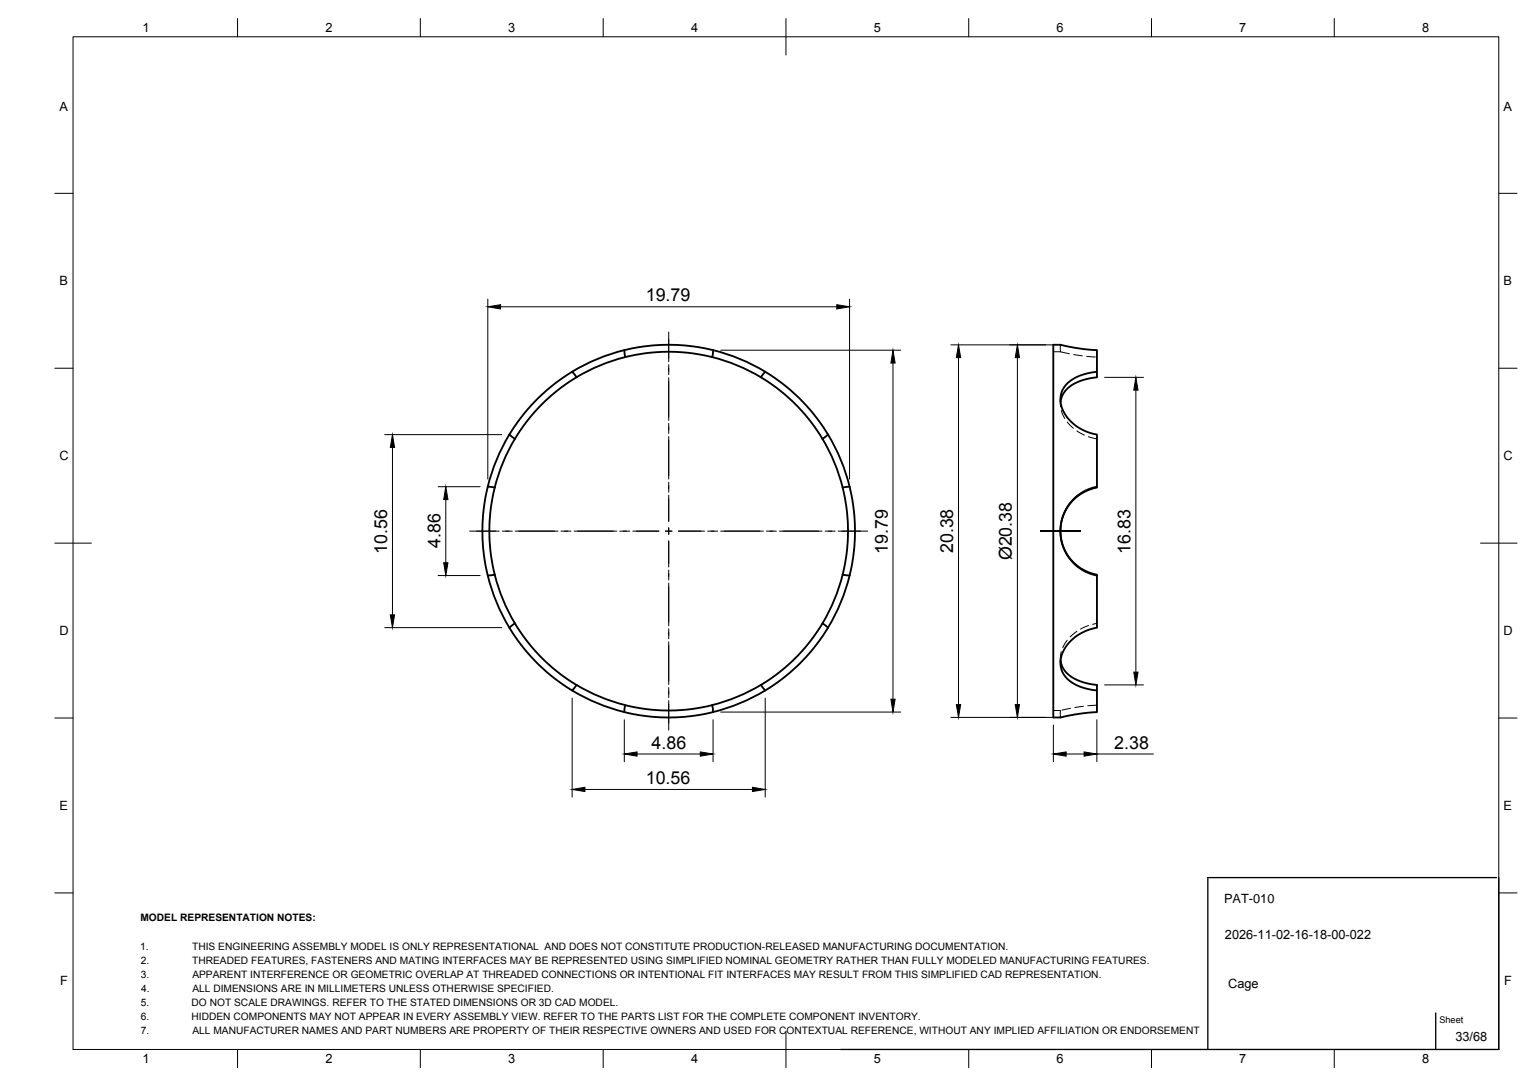
ISO-10303-21;
HEADER;
/* Generated by software containing ST-Developer
 * from STEP Tools, Inc. (www.steptools.com) 
 */

FILE_DESCRIPTION(
/* description */ ('Belt conveyor head drive unit'),
/* implementation_level */ '2;1');

FILE_NAME(
/* name */ 'Cage.step',
/* time_stamp */ '2026-10-28T03:26:19-07:00',
/* author */ (''),
/* organization */ (''),
/* preprocessor_version */ 'ST-DEVELOPER v20.2',
/* originating_system */ 'Autodesk Translation Framework v15.17.0.0',
/* authorisation */ '');

FILE_SCHEMA (('AUTOMOTIVE_DESIGN { 1 0 10303 214 3 1 1 }'));
ENDSEC;

DATA;
#10=MECHANICAL_DESIGN_GEOMETRIC_PRESENTATION_REPRESENTATION('',(#884),#27069);
#521=B_SPLINE_CURVE_WITH_KNOTS('',3,(#22504,#22505,#22506,#22507,#22508,
#22509,#22510,#22511,#22512,#22513,#22514,#22515,#22516,#22517,#22518,#22519,
#22520,#22521,#22522,#22523,#22524,#22525),.UNSPECIFIED.,.F.,.F.,(4,2,2,
2,2,2,2,2,2,2,4),(0.0473477652366656,0.126350602536658,0.189525903804987,
0.252701205073317,0.313298422430275,0.373895639787233,0.434492857144191,
0.495090074501149,0.558265375769478,0.621440677037807,0.7004435143378),
 .UNSPECIFIED.);
#522=B_SPLINE_CURVE_WITH_KNOTS('',3,(#22529,#22530,#22531,#22532,#22533,
#22534,#22535,#22536,#22537,#22538,#22539,#22540,#22541,#22542,#22543,#22544,
#22545,#22546,#22547,#22548,#22549,#22550),.UNSPECIFIED.,.F.,.F.,(4,2,2,
2,2,2,2,2,2,2,4),(0.0464897534940957,0.0852567806515119,0.170513561303024,
0.246687263103517,0.308657850341199,0.370628437578881,0.432599024816563,
0.494569612054245,0.570743313854739,0.656000094506251,0.694767121663666),
 .UNSPECIFIED.);
#523=B_SPLINE_CURVE_WITH_KNOTS('',3,(#22556,#22557,#22558,#22559,#22560,
#22561,#22562,#22563,#22564,#22565,#22566,#22567,#22568,#22569,#22570,#22571,
#22572,#22573,#22574,#22575,#22576,#22577),.UNSPECIFIED.,.F.,.F.,(4,2,2,
2,2,2,2,2,2,2,4),(0.0464897534940957,0.0852567806515118,0.170513561303024,
0.246687263103517,0.308657850341199,0.370628437578881,0.432599024816563,
0.494569612054245,0.570743313854738,0.65600009450625,0.694767121663666),
 .UNSPECIFIED.);
#524=B_SPLINE_CURVE_WITH_KNOTS('',3,(#22581,#22582,#22583,#22584,#22585,
#22586,#22587,#22588,#22589,#22590,#22591,#22592,#22593,#22594,#22595,#22596,
#22597,#22598,#22599,#22600,#22601,#22602),.UNSPECIFIED.,.F.,.F.,(4,2,2,
2,2,2,2,2,2,2,4),(0.0464897534940957,0.0852567806515119,0.170513561303024,
0.246687263103517,0.308657850341199,0.370628437578881,0.432599024816563,
0.494569612054245,0.570743313854739,0.656000094506251,0.694767121663666),
 .UNSPECIFIED.);
#525=B_SPLINE_CURVE_WITH_KNOTS('',3,(#22606,#22607,#22608,#22609,#22610,
#22611,#22612,#22613,#22614,#22615,#22616,#22617),.UNSPECIFIED.,.F.,.F.,
(4,2,2,2,2,4),(0.0464897534940957,0.0852567806515119,0.170513561303024,
0.246687263103517,0.308657850341199,0.370628437578881),.UNSPECIFIED.);
#526=B_SPLINE_CURVE_WITH_KNOTS('',3,(#22622,#22623,#22624,#22625,#22626,
#22627,#22628,#22629,#22630,#22631,#22632,#22633),.UNSPECIFIED.,.F.,.F.,
(4,2,2,2,2,4),(0.370628437578881,0.432599024816563,0.494569612054245,0.570743313854738,
0.65600009450625,0.694767121663666),.UNSPECIFIED.);
#527=B_SPLINE_CURVE_WITH_KNOTS('',3,(#22637,#22638,#22639,#22640,#22641,
#22642,#22643,#22644,#22645,#22646,#22647,#22648,#22649,#22650,#22651,#22652,
#22653,#22654,#22655,#22656,#22657,#22658),.UNSPECIFIED.,.F.,.F.,(4,2,2,
2,2,2,2,2,2,2,4),(0.0464897534940957,0.0852567806515121,0.170513561303024,
0.246687263103518,0.308657850341199,0.370628437578881,0.432599024816563,
0.494569612054245,0.570743313854738,0.65600009450625,0.694767121663666),
 .UNSPECIFIED.);
#528=B_SPLINE_CURVE_WITH_KNOTS('',3,(#22662,#22663,#22664,#22665,#22666,
#22667,#22668,#22669,#22670,#22671,#22672,#22673,#22674,#22675,#22676,#22677,
#22678,#22679,#22680,#22681,#22682,#22683),.UNSPECIFIED.,.F.,.F.,(4,2,2,
2,2,2,2,2,2,2,4),(0.0464897534940957,0.0852567806515119,0.170513561303024,
0.246687263103517,0.308657850341199,0.370628437578881,0.432599024816563,
0.494569612054245,0.570743313854738,0.65600009450625,0.694767121663667),
 .UNSPECIFIED.);
#529=B_SPLINE_CURVE_WITH_KNOTS('',3,(#22687,#22688,#22689,#22690,#22691,
#22692,#22693,#22694,#22695,#22696,#22697,#22698,#22699,#22700,#22701,#22702,
#22703,#22704,#22705,#22706,#22707,#22708),.UNSPECIFIED.,.F.,.F.,(4,2,2,
2,2,2,2,2,2,2,4),(0.0464897534940957,0.0852567806515119,0.170513561303024,
0.246687263103517,0.308657850341199,0.370628437578881,0.432599024816563,
0.494569612054245,0.570743313854738,0.65600009450625,0.694767121663666),
 .UNSPECIFIED.);
#530=B_SPLINE_CURVE_WITH_KNOTS('',3,(#22712,#22713,#22714,#22715,#22716,
#22717,#22718,#22719,#22720,#22721,#22722,#22723,#22724,#22725,#22726,#22727,
#22728,#22729,#22730,#22731,#22732,#22733),.UNSPECIFIED.,.F.,.F.,(4,2,2,
2,2,2,2,2,2,2,4),(0.0464897534940957,0.0852567806515119,0.170513561303024,
0.246687263103517,0.308657850341199,0.370628437578881,0.432599024816563,
0.494569612054245,0.570743313854739,0.656000094506251,0.694767121663667),
 .UNSPECIFIED.);
#531=B_SPLINE_CURVE_WITH_KNOTS('',3,(#22741,#22742,#22743,#22744,#22745,
#22746,#22747,#22748,#22749,#22750,#22751,#22752,#22753,#22754,#22755,#22756,
#22757,#22758,#22759,#22760,#22761,#22762),.UNSPECIFIED.,.F.,.F.,(4,2,2,
2,2,2,2,2,2,2,4),(0.0473477652366656,0.126350602536658,0.189525903804987,
0.252701205073316,0.313298422430274,0.373895639787232,0.434492857144191,
0.495090074501149,0.558265375769478,0.621440677037807,0.7004435143378),
 .UNSPECIFIED.);
#532=B_SPLINE_CURVE_WITH_KNOTS('',3,(#22770,#22771,#22772,#22773,#22774,
#22775,#22776,#22777,#22778,#22779,#22780,#22781,#22782,#22783,#22784,#22785,
#22786,#22787,#22788,#22789,#22790,#22791),.UNSPECIFIED.,.F.,.F.,(4,2,2,
2,2,2,2,2,2,2,4),(0.0473477652366656,0.126350602536658,0.189525903804987,
0.252701205073317,0.313298422430275,0.373895639787233,0.434492857144191,
0.495090074501149,0.558265375769478,0.621440677037807,0.7004435143378),
 .UNSPECIFIED.);
#533=B_SPLINE_CURVE_WITH_KNOTS('',3,(#22800,#22801,#22802,#22803,#22804,
#22805,#22806,#22807,#22808,#22809,#22810,#22811),.UNSPECIFIED.,.F.,.F.,
(4,2,2,2,2,4),(0.0473477652366656,0.126350602536658,0.189525903804987,0.252701205073316,
0.313298422430275,0.373895639787233),.UNSPECIFIED.);
#534=B_SPLINE_CURVE_WITH_KNOTS('',3,(#22813,#22814,#22815,#22816,#22817,
#22818,#22819,#22820,#22821,#22822,#22823,#22824),.UNSPECIFIED.,.F.,.F.,
(4,2,2,2,2,4),(0.373895639787233,0.434492857144191,0.495090074501149,0.558265375769478,
0.621440677037807,0.7004435143378),.UNSPECIFIED.);
#535=B_SPLINE_CURVE_WITH_KNOTS('',3,(#22831,#22832,#22833,#22834,#22835,
#22836,#22837,#22838,#22839,#22840,#22841,#22842,#22843,#22844,#22845,#22846,
#22847,#22848,#22849,#22850,#22851,#22852),.UNSPECIFIED.,.F.,.F.,(4,2,2,
2,2,2,2,2,2,2,4),(0.0473477652366656,0.126350602536658,0.189525903804987,
0.252701205073316,0.313298422430275,0.373895639787233,0.434492857144191,
0.495090074501149,0.558265375769478,0.621440677037807,0.7004435143378),
 .UNSPECIFIED.);
#536=B_SPLINE_CURVE_WITH_KNOTS('',3,(#22860,#22861,#22862,#22863,#22864,
#22865,#22866,#22867,#22868,#22869,#22870,#22871,#22872,#22873,#22874,#22875,
#22876,#22877,#22878,#22879,#22880,#22881),.UNSPECIFIED.,.F.,.F.,(4,2,2,
2,2,2,2,2,2,2,4),(0.0473477652366656,0.126350602536658,0.189525903804987,
0.252701205073317,0.313298422430275,0.373895639787233,0.434492857144191,
0.495090074501149,0.558265375769478,0.621440677037807,0.7004435143378),
 .UNSPECIFIED.);
#537=B_SPLINE_CURVE_WITH_KNOTS('',3,(#22889,#22890,#22891,#22892,#22893,
#22894,#22895,#22896,#22897,#22898,#22899,#22900,#22901,#22902,#22903,#22904,
#22905,#22906,#22907,#22908,#22909,#22910),.UNSPECIFIED.,.F.,.F.,(4,2,2,
2,2,2,2,2,2,2,4),(0.0473477652366656,0.126350602536658,0.189525903804987,
0.252701205073316,0.313298422430275,0.373895639787233,0.434492857144191,
0.495090074501149,0.558265375769478,0.621440677037807,0.7004435143378),
 .UNSPECIFIED.);
#538=B_SPLINE_CURVE_WITH_KNOTS('',3,(#22919,#22920,#22921,#22922,#22923,
#22924,#22925,#22926,#22927,#22928,#22929,#22930,#22931,#22932,#22933,#22934,
#22935,#22936,#22937,#22938,#22939,#22940),.UNSPECIFIED.,.F.,.F.,(4,2,2,
2,2,2,2,2,2,2,4),(0.0473477652366656,0.126350602536658,0.189525903804987,
0.252701205073317,0.313298422430275,0.373895639787233,0.434492857144191,
0.495090074501149,0.558265375769478,0.621440677037807,0.7004435143378),
 .UNSPECIFIED.);
#653=SPHERICAL_SURFACE('',#15248,0.247676);
#654=SPHERICAL_SURFACE('',#15264,0.247676);
#655=SPHERICAL_SURFACE('',#15269,0.247676);
#656=SPHERICAL_SURFACE('',#15274,0.247676);
#657=SPHERICAL_SURFACE('',#15279,0.247676);
#658=SPHERICAL_SURFACE('',#15284,0.247676);
#659=SPHERICAL_SURFACE('',#15289,0.247676);
#660=SPHERICAL_SURFACE('',#15297,0.247676);
#739=SHAPE_REPRESENTATION_RELATIONSHIP('SRR','None',#27384,#808);
#808=ADVANCED_BREP_SHAPE_REPRESENTATION('',(#969),#27026);
#884=STYLED_ITEM('',(#27797),#969);
#969=MANIFOLD_SOLID_BREP('Continuous crown cage',#13749);
#1155=FACE_BOUND('',#2920,.T.);
#1441=PLANE('',#15261);
#1442=PLANE('',#15266);
#1443=PLANE('',#15271);
#1444=PLANE('',#15276);
#1445=PLANE('',#15281);
#1446=PLANE('',#15286);
#1447=PLANE('',#15295);
#1448=PLANE('',#15299);
#1449=PLANE('',#15300);
#1959=FACE_OUTER_BOUND('',#2902,.T.);
#1960=FACE_OUTER_BOUND('',#2903,.T.);
#1961=FACE_OUTER_BOUND('',#2904,.T.);
#1962=FACE_OUTER_BOUND('',#2905,.T.);
#1963=FACE_OUTER_BOUND('',#2906,.T.);
#1964=FACE_OUTER_BOUND('',#2907,.T.);
#1965=FACE_OUTER_BOUND('',#2908,.T.);
#1966=FACE_OUTER_BOUND('',#2909,.T.);
#1967=FACE_OUTER_BOUND('',#2910,.T.);
#1968=FACE_OUTER_BOUND('',#2911,.T.);
#1969=FACE_OUTER_BOUND('',#2912,.T.);
#1970=FACE_OUTER_BOUND('',#2913,.T.);
#1971=FACE_OUTER_BOUND('',#2914,.T.);
#1972=FACE_OUTER_BOUND('',#2915,.T.);
#1973=FACE_OUTER_BOUND('',#2916,.T.);
#1974=FACE_OUTER_BOUND('',#2917,.T.);
#1975=FACE_OUTER_BOUND('',#2918,.T.);
#1976=FACE_OUTER_BOUND('',#2919,.T.);
#1977=FACE_OUTER_BOUND('',#2921,.T.);
#2902=EDGE_LOOP('',(#10352,#10353,#10354,#10355));
#2903=EDGE_LOOP('',(#10356,#10357,#10358,#10359,#10360,#10361,#10362,#10363,
#10364,#10365,#10366,#10367,#10368,#10369,#10370,#10371,#10372,#10373,#10374,
#10375));
#2904=EDGE_LOOP('',(#10376,#10377,#10378,#10379));
#2905=EDGE_LOOP('',(#10380,#10381,#10382,#10383));
#2906=EDGE_LOOP('',(#10384,#10385,#10386,#10387));
#2907=EDGE_LOOP('',(#10388,#10389,#10390,#10391));
#2908=EDGE_LOOP('',(#10392,#10393,#10394,#10395));
#2909=EDGE_LOOP('',(#10396,#10397,#10398,#10399,#10400,#10401));
#2910=EDGE_LOOP('',(#10402,#10403,#10404,#10405));
#2911=EDGE_LOOP('',(#10406,#10407,#10408,#10409));
#2912=EDGE_LOOP('',(#10410,#10411,#10412,#10413));
#2913=EDGE_LOOP('',(#10414,#10415,#10416,#10417));
#2914=EDGE_LOOP('',(#10418,#10419,#10420,#10421));
#2915=EDGE_LOOP('',(#10422,#10423,#10424,#10425));
#2916=EDGE_LOOP('',(#10426,#10427,#10428,#10429,#10430,#10431,#10432,#10433,
#10434,#10435,#10436,#10437,#10438,#10439,#10440,#10441,#10442,#10443,#10444,
#10445));
#2917=EDGE_LOOP('',(#10446,#10447,#10448,#10449));
#2918=EDGE_LOOP('',(#10450,#10451,#10452,#10453));
#2919=EDGE_LOOP('',(#10454));
#2920=EDGE_LOOP('',(#10455));
#2921=EDGE_LOOP('',(#10456,#10457,#10458,#10459));
#3869=LINE('',#22619,#4661);
#3870=LINE('',#22915,#4662);
#4661=VECTOR('',#18191,1.019052);
#4662=VECTOR('',#18268,0.980948);
#5408=CIRCLE('',#15249,0.243053047864041);
#5409=CIRCLE('',#15250,0.243053047864041);
#5410=CIRCLE('',#15252,1.019052);
#5411=CIRCLE('',#15253,1.019052);
#5412=CIRCLE('',#15254,1.019052);
#5413=CIRCLE('',#15255,1.019052);
#5414=CIRCLE('',#15256,1.019052);
#5415=CIRCLE('',#15257,1.019052);
#5416=CIRCLE('',#15258,1.019052);
#5417=CIRCLE('',#15259,1.019052);
#5418=CIRCLE('',#15260,1.019052);
#5419=CIRCLE('',#15262,0.980948);
#5420=CIRCLE('',#15263,0.243053047864041);
#5421=CIRCLE('',#15265,0.243053047864041);
#5422=CIRCLE('',#15267,0.980948);
#5423=CIRCLE('',#15268,0.243053047864041);
#5424=CIRCLE('',#15270,0.243053047864041);
#5425=CIRCLE('',#15272,0.980948);
#5426=CIRCLE('',#15273,0.243053047864041);
#5427=CIRCLE('',#15275,0.243053047864041);
#5428=CIRCLE('',#15277,0.980948);
#5429=CIRCLE('',#15278,0.243053047864041);
#5430=CIRCLE('',#15280,0.243053047864041);
#5431=CIRCLE('',#15282,0.980948);
#5432=CIRCLE('',#15283,0.243053047864041);
#5433=CIRCLE('',#15285,0.243053047864041);
#5434=CIRCLE('',#15287,0.980948);
#5435=CIRCLE('',#15288,0.243053047864041);
#5436=CIRCLE('',#15290,0.243053047864041);
#5437=CIRCLE('',#15292,0.980948);
#5438=CIRCLE('',#15293,0.980948);
#5439=CIRCLE('',#15294,0.980948);
#5440=CIRCLE('',#15296,0.243053047864041);
#5441=CIRCLE('',#15298,0.243053047864041);
#6427=VERTEX_POINT('',#22502);
#6428=VERTEX_POINT('',#22503);
#6429=VERTEX_POINT('',#22526);
#6430=VERTEX_POINT('',#22528);
#6431=VERTEX_POINT('',#22553);
#6432=VERTEX_POINT('',#22555);
#6433=VERTEX_POINT('',#22578);
#6434=VERTEX_POINT('',#22580);
#6435=VERTEX_POINT('',#22603);
#6436=VERTEX_POINT('',#22605);
#6437=VERTEX_POINT('',#22618);
#6438=VERTEX_POINT('',#22621);
#6439=VERTEX_POINT('',#22634);
#6440=VERTEX_POINT('',#22636);
#6441=VERTEX_POINT('',#22659);
#6442=VERTEX_POINT('',#22661);
#6443=VERTEX_POINT('',#22684);
#6444=VERTEX_POINT('',#22686);
#6445=VERTEX_POINT('',#22709);
#6446=VERTEX_POINT('',#22711);
#6447=VERTEX_POINT('',#22736);
#6448=VERTEX_POINT('',#22740);
#6449=VERTEX_POINT('',#22765);
#6450=VERTEX_POINT('',#22769);
#6451=VERTEX_POINT('',#22794);
#6452=VERTEX_POINT('',#22798);
#6453=VERTEX_POINT('',#22799);
#6454=VERTEX_POINT('',#22826);
#6455=VERTEX_POINT('',#22830);
#6456=VERTEX_POINT('',#22855);
#6457=VERTEX_POINT('',#22859);
#6458=VERTEX_POINT('',#22884);
#6459=VERTEX_POINT('',#22888);
#6460=VERTEX_POINT('',#22913);
#6461=VERTEX_POINT('',#22916);
#6462=VERTEX_POINT('',#22918);
#7868=EDGE_CURVE('',#6427,#6428,#521,.T.);
#7869=EDGE_CURVE('',#6429,#6427,#5408,.T.);
#7870=EDGE_CURVE('',#6430,#6429,#522,.T.);
#7871=EDGE_CURVE('',#6428,#6430,#5409,.T.);
#7872=EDGE_CURVE('',#6431,#6429,#5410,.T.);
#7873=EDGE_CURVE('',#6431,#6432,#523,.T.);
#7874=EDGE_CURVE('',#6433,#6432,#5411,.T.);
#7875=EDGE_CURVE('',#6433,#6434,#524,.T.);
#7876=EDGE_CURVE('',#6435,#6434,#5412,.T.);
#7877=EDGE_CURVE('',#6435,#6436,#525,.T.);
#7878=EDGE_CURVE('',#6436,#6437,#3869,.T.);
#7879=EDGE_CURVE('',#6437,#6437,#5413,.T.);
#7880=EDGE_CURVE('',#6436,#6438,#526,.T.);
#7881=EDGE_CURVE('',#6439,#6438,#5414,.T.);
#7882=EDGE_CURVE('',#6439,#6440,#527,.T.);
#7883=EDGE_CURVE('',#6441,#6440,#5415,.T.);
#7884=EDGE_CURVE('',#6441,#6442,#528,.T.);
#7885=EDGE_CURVE('',#6443,#6442,#5416,.T.);
#7886=EDGE_CURVE('',#6443,#6444,#529,.T.);
#7887=EDGE_CURVE('',#6445,#6444,#5417,.T.);
#7888=EDGE_CURVE('',#6445,#6446,#530,.T.);
#7889=EDGE_CURVE('',#6430,#6446,#5418,.T.);
#7890=EDGE_CURVE('',#6427,#6447,#5419,.T.);
#7891=EDGE_CURVE('',#6447,#6431,#5420,.T.);
#7892=EDGE_CURVE('',#6448,#6447,#531,.T.);
#7893=EDGE_CURVE('',#6432,#6448,#5421,.T.);
#7894=EDGE_CURVE('',#6448,#6449,#5422,.T.);
#7895=EDGE_CURVE('',#6449,#6433,#5423,.T.);
#7896=EDGE_CURVE('',#6450,#6449,#532,.T.);
#7897=EDGE_CURVE('',#6434,#6450,#5424,.T.);
#7898=EDGE_CURVE('',#6450,#6451,#5425,.T.);
#7899=EDGE_CURVE('',#6451,#6435,#5426,.T.);
#7900=EDGE_CURVE('',#6452,#6453,#533,.T.);
#7901=EDGE_CURVE('',#6438,#6452,#5427,.T.);
#7902=EDGE_CURVE('',#6453,#6451,#534,.T.);
#7903=EDGE_CURVE('',#6452,#6454,#5428,.T.);
#7904=EDGE_CURVE('',#6454,#6439,#5429,.T.);
#7905=EDGE_CURVE('',#6455,#6454,#535,.T.);
#7906=EDGE_CURVE('',#6440,#6455,#5430,.T.);
#7907=EDGE_CURVE('',#6455,#6456,#5431,.T.);
#7908=EDGE_CURVE('',#6456,#6441,#5432,.T.);
#7909=EDGE_CURVE('',#6457,#6456,#536,.T.);
#7910=EDGE_CURVE('',#6442,#6457,#5433,.T.);
#7911=EDGE_CURVE('',#6457,#6458,#5434,.T.);
#7912=EDGE_CURVE('',#6458,#6443,#5435,.T.);
#7913=EDGE_CURVE('',#6459,#6458,#537,.T.);
#7914=EDGE_CURVE('',#6444,#6459,#5436,.T.);
#7915=EDGE_CURVE('',#6460,#6460,#5437,.T.);
#7916=EDGE_CURVE('',#6460,#6453,#3870,.T.);
#7917=EDGE_CURVE('',#6461,#6428,#5438,.T.);
#7918=EDGE_CURVE('',#6461,#6462,#538,.T.);
#7919=EDGE_CURVE('',#6459,#6462,#5439,.T.);
#7920=EDGE_CURVE('',#6446,#6461,#5440,.T.);
#7921=EDGE_CURVE('',#6462,#6445,#5441,.T.);
#10352=ORIENTED_EDGE('',*,*,#7868,.F.);
#10353=ORIENTED_EDGE('',*,*,#7869,.F.);
#10354=ORIENTED_EDGE('',*,*,#7870,.F.);
#10355=ORIENTED_EDGE('',*,*,#7871,.F.);
#10356=ORIENTED_EDGE('',*,*,#7870,.T.);
#10357=ORIENTED_EDGE('',*,*,#7872,.F.);
#10358=ORIENTED_EDGE('',*,*,#7873,.T.);
#10359=ORIENTED_EDGE('',*,*,#7874,.F.);
#10360=ORIENTED_EDGE('',*,*,#7875,.T.);
#10361=ORIENTED_EDGE('',*,*,#7876,.F.);
#10362=ORIENTED_EDGE('',*,*,#7877,.T.);
#10363=ORIENTED_EDGE('',*,*,#7878,.T.);
#10364=ORIENTED_EDGE('',*,*,#7879,.F.);
#10365=ORIENTED_EDGE('',*,*,#7878,.F.);
#10366=ORIENTED_EDGE('',*,*,#7880,.T.);
#10367=ORIENTED_EDGE('',*,*,#7881,.F.);
#10368=ORIENTED_EDGE('',*,*,#7882,.T.);
#10369=ORIENTED_EDGE('',*,*,#7883,.F.);
#10370=ORIENTED_EDGE('',*,*,#7884,.T.);
#10371=ORIENTED_EDGE('',*,*,#7885,.F.);
#10372=ORIENTED_EDGE('',*,*,#7886,.T.);
#10373=ORIENTED_EDGE('',*,*,#7887,.F.);
#10374=ORIENTED_EDGE('',*,*,#7888,.T.);
#10375=ORIENTED_EDGE('',*,*,#7889,.F.);
#10376=ORIENTED_EDGE('',*,*,#7869,.T.);
#10377=ORIENTED_EDGE('',*,*,#7890,.T.);
#10378=ORIENTED_EDGE('',*,*,#7891,.T.);
#10379=ORIENTED_EDGE('',*,*,#7872,.T.);
#10380=ORIENTED_EDGE('',*,*,#7892,.F.);
#10381=ORIENTED_EDGE('',*,*,#7893,.F.);
#10382=ORIENTED_EDGE('',*,*,#7873,.F.);
#10383=ORIENTED_EDGE('',*,*,#7891,.F.);
#10384=ORIENTED_EDGE('',*,*,#7893,.T.);
#10385=ORIENTED_EDGE('',*,*,#7894,.T.);
#10386=ORIENTED_EDGE('',*,*,#7895,.T.);
#10387=ORIENTED_EDGE('',*,*,#7874,.T.);
#10388=ORIENTED_EDGE('',*,*,#7896,.F.);
#10389=ORIENTED_EDGE('',*,*,#7897,.F.);
#10390=ORIENTED_EDGE('',*,*,#7875,.F.);
#10391=ORIENTED_EDGE('',*,*,#7895,.F.);
#10392=ORIENTED_EDGE('',*,*,#7897,.T.);
#10393=ORIENTED_EDGE('',*,*,#7898,.T.);
#10394=ORIENTED_EDGE('',*,*,#7899,.T.);
#10395=ORIENTED_EDGE('',*,*,#7876,.T.);
#10396=ORIENTED_EDGE('',*,*,#7900,.F.);
#10397=ORIENTED_EDGE('',*,*,#7901,.F.);
#10398=ORIENTED_EDGE('',*,*,#7880,.F.);
#10399=ORIENTED_EDGE('',*,*,#7877,.F.);
#10400=ORIENTED_EDGE('',*,*,#7899,.F.);
#10401=ORIENTED_EDGE('',*,*,#7902,.F.);
#10402=ORIENTED_EDGE('',*,*,#7901,.T.);
#10403=ORIENTED_EDGE('',*,*,#7903,.T.);
#10404=ORIENTED_EDGE('',*,*,#7904,.T.);
#10405=ORIENTED_EDGE('',*,*,#7881,.T.);
#10406=ORIENTED_EDGE('',*,*,#7905,.F.);
#10407=ORIENTED_EDGE('',*,*,#7906,.F.);
#10408=ORIENTED_EDGE('',*,*,#7882,.F.);
#10409=ORIENTED_EDGE('',*,*,#7904,.F.);
#10410=ORIENTED_EDGE('',*,*,#7906,.T.);
#10411=ORIENTED_EDGE('',*,*,#7907,.T.);
#10412=ORIENTED_EDGE('',*,*,#7908,.T.);
#10413=ORIENTED_EDGE('',*,*,#7883,.T.);
#10414=ORIENTED_EDGE('',*,*,#7909,.F.);
#10415=ORIENTED_EDGE('',*,*,#7910,.F.);
#10416=ORIENTED_EDGE('',*,*,#7884,.F.);
#10417=ORIENTED_EDGE('',*,*,#7908,.F.);
#10418=ORIENTED_EDGE('',*,*,#7910,.T.);
#10419=ORIENTED_EDGE('',*,*,#7911,.T.);
#10420=ORIENTED_EDGE('',*,*,#7912,.T.);
#10421=ORIENTED_EDGE('',*,*,#7885,.T.);
#10422=ORIENTED_EDGE('',*,*,#7886,.F.);
#10423=ORIENTED_EDGE('',*,*,#7912,.F.);
#10424=ORIENTED_EDGE('',*,*,#7913,.F.);
#10425=ORIENTED_EDGE('',*,*,#7914,.F.);
#10426=ORIENTED_EDGE('',*,*,#7915,.F.);
#10427=ORIENTED_EDGE('',*,*,#7916,.T.);
#10428=ORIENTED_EDGE('',*,*,#7902,.T.);
#10429=ORIENTED_EDGE('',*,*,#7898,.F.);
#10430=ORIENTED_EDGE('',*,*,#7896,.T.);
#10431=ORIENTED_EDGE('',*,*,#7894,.F.);
#10432=ORIENTED_EDGE('',*,*,#7892,.T.);
#10433=ORIENTED_EDGE('',*,*,#7890,.F.);
#10434=ORIENTED_EDGE('',*,*,#7868,.T.);
#10435=ORIENTED_EDGE('',*,*,#7917,.F.);
#10436=ORIENTED_EDGE('',*,*,#7918,.T.);
#10437=ORIENTED_EDGE('',*,*,#7919,.F.);
#10438=ORIENTED_EDGE('',*,*,#7913,.T.);
#10439=ORIENTED_EDGE('',*,*,#7911,.F.);
#10440=ORIENTED_EDGE('',*,*,#7909,.T.);
#10441=ORIENTED_EDGE('',*,*,#7907,.F.);
#10442=ORIENTED_EDGE('',*,*,#7905,.T.);
#10443=ORIENTED_EDGE('',*,*,#7903,.F.);
#10444=ORIENTED_EDGE('',*,*,#7900,.T.);
#10445=ORIENTED_EDGE('',*,*,#7916,.F.);
#10446=ORIENTED_EDGE('',*,*,#7871,.T.);
#10447=ORIENTED_EDGE('',*,*,#7889,.T.);
#10448=ORIENTED_EDGE('',*,*,#7920,.T.);
#10449=ORIENTED_EDGE('',*,*,#7917,.T.);
#10450=ORIENTED_EDGE('',*,*,#7888,.F.);
#10451=ORIENTED_EDGE('',*,*,#7921,.F.);
#10452=ORIENTED_EDGE('',*,*,#7918,.F.);
#10453=ORIENTED_EDGE('',*,*,#7920,.F.);
#10454=ORIENTED_EDGE('',*,*,#7879,.T.);
#10455=ORIENTED_EDGE('',*,*,#7915,.T.);
#10456=ORIENTED_EDGE('',*,*,#7914,.T.);
#10457=ORIENTED_EDGE('',*,*,#7919,.T.);
#10458=ORIENTED_EDGE('',*,*,#7921,.T.);
#10459=ORIENTED_EDGE('',*,*,#7887,.T.);
#12680=CYLINDRICAL_SURFACE('',#15251,1.019052);
#12681=CYLINDRICAL_SURFACE('',#15291,0.980948);
#13238=ADVANCED_FACE('',(#1959),#653,.F.);
#13239=ADVANCED_FACE('',(#1960),#12680,.T.);
#13240=ADVANCED_FACE('',(#1961),#1441,.T.);
#13241=ADVANCED_FACE('',(#1962),#654,.F.);
#13242=ADVANCED_FACE('',(#1963),#1442,.T.);
#13243=ADVANCED_FACE('',(#1964),#655,.F.);
#13244=ADVANCED_FACE('',(#1965),#1443,.T.);
#13245=ADVANCED_FACE('',(#1966),#656,.F.);
#13246=ADVANCED_FACE('',(#1967),#1444,.T.);
#13247=ADVANCED_FACE('',(#1968),#657,.F.);
#13248=ADVANCED_FACE('',(#1969),#1445,.T.);
#13249=ADVANCED_FACE('',(#1970),#658,.F.);
#13250=ADVANCED_FACE('',(#1971),#1446,.T.);
#13251=ADVANCED_FACE('',(#1972),#659,.F.);
#13252=ADVANCED_FACE('',(#1973),#12681,.F.);
#13253=ADVANCED_FACE('',(#1974),#1447,.T.);
#13254=ADVANCED_FACE('',(#1975),#660,.F.);
#13255=ADVANCED_FACE('',(#1976,#1155),#1448,.T.);
#13256=ADVANCED_FACE('',(#1977),#1449,.T.);
#13749=CLOSED_SHELL('',(#13238,#13239,#13240,#13241,#13242,#13243,#13244,
#13245,#13246,#13247,#13248,#13249,#13250,#13251,#13252,#13253,#13254,#13255,
#13256));
#15247=AXIS2_PLACEMENT_3D('',#22500,#18175,#18176);
#15248=AXIS2_PLACEMENT_3D('',#22501,#18177,#18178);
#15249=AXIS2_PLACEMENT_3D('',#22527,#18179,#18180);
#15250=AXIS2_PLACEMENT_3D('',#22551,#18181,#18182);
#15251=AXIS2_PLACEMENT_3D('',#22552,#18183,#18184);
#15252=AXIS2_PLACEMENT_3D('',#22554,#18185,#18186);
#15253=AXIS2_PLACEMENT_3D('',#22579,#18187,#18188);
#15254=AXIS2_PLACEMENT_3D('',#22604,#18189,#18190);
#15255=AXIS2_PLACEMENT_3D('',#22620,#18192,#18193);
#15256=AXIS2_PLACEMENT_3D('',#22635,#18194,#18195);
#15257=AXIS2_PLACEMENT_3D('',#22660,#18196,#18197);
#15258=AXIS2_PLACEMENT_3D('',#22685,#18198,#18199);
#15259=AXIS2_PLACEMENT_3D('',#22710,#18200,#18201);
#15260=AXIS2_PLACEMENT_3D('',#22734,#18202,#18203);
#15261=AXIS2_PLACEMENT_3D('',#22735,#18204,#18205);
#15262=AXIS2_PLACEMENT_3D('',#22737,#18206,#18207);
#15263=AXIS2_PLACEMENT_3D('',#22738,#18208,#18209);
#15264=AXIS2_PLACEMENT_3D('',#22739,#18210,#18211);
#15265=AXIS2_PLACEMENT_3D('',#22763,#18212,#18213);
#15266=AXIS2_PLACEMENT_3D('',#22764,#18214,#18215);
#15267=AXIS2_PLACEMENT_3D('',#22766,#18216,#18217);
#15268=AXIS2_PLACEMENT_3D('',#22767,#18218,#18219);
#15269=AXIS2_PLACEMENT_3D('',#22768,#18220,#18221);
#15270=AXIS2_PLACEMENT_3D('',#22792,#18222,#18223);
#15271=AXIS2_PLACEMENT_3D('',#22793,#18224,#18225);
#15272=AXIS2_PLACEMENT_3D('',#22795,#18226,#18227);
#15273=AXIS2_PLACEMENT_3D('',#22796,#18228,#18229);
#15274=AXIS2_PLACEMENT_3D('',#22797,#18230,#18231);
#15275=AXIS2_PLACEMENT_3D('',#22812,#18232,#18233);
#15276=AXIS2_PLACEMENT_3D('',#22825,#18234,#18235);
#15277=AXIS2_PLACEMENT_3D('',#22827,#18236,#18237);
#15278=AXIS2_PLACEMENT_3D('',#22828,#18238,#18239);
#15279=AXIS2_PLACEMENT_3D('',#22829,#18240,#18241);
#15280=AXIS2_PLACEMENT_3D('',#22853,#18242,#18243);
#15281=AXIS2_PLACEMENT_3D('',#22854,#18244,#18245);
#15282=AXIS2_PLACEMENT_3D('',#22856,#18246,#18247);
#15283=AXIS2_PLACEMENT_3D('',#22857,#18248,#18249);
#15284=AXIS2_PLACEMENT_3D('',#22858,#18250,#18251);
#15285=AXIS2_PLACEMENT_3D('',#22882,#18252,#18253);
#15286=AXIS2_PLACEMENT_3D('',#22883,#18254,#18255);
#15287=AXIS2_PLACEMENT_3D('',#22885,#18256,#18257);
#15288=AXIS2_PLACEMENT_3D('',#22886,#18258,#18259);
#15289=AXIS2_PLACEMENT_3D('',#22887,#18260,#18261);
#15290=AXIS2_PLACEMENT_3D('',#22911,#18262,#18263);
#15291=AXIS2_PLACEMENT_3D('',#22912,#18264,#18265);
#15292=AXIS2_PLACEMENT_3D('',#22914,#18266,#18267);
#15293=AXIS2_PLACEMENT_3D('',#22917,#18269,#18270);
#15294=AXIS2_PLACEMENT_3D('',#22941,#18271,#18272);
#15295=AXIS2_PLACEMENT_3D('',#22942,#18273,#18274);
#15296=AXIS2_PLACEMENT_3D('',#22943,#18275,#18276);
#15297=AXIS2_PLACEMENT_3D('',#22944,#18277,#18278);
#15298=AXIS2_PLACEMENT_3D('',#22945,#18279,#18280);
#15299=AXIS2_PLACEMENT_3D('',#22946,#18281,#18282);
#15300=AXIS2_PLACEMENT_3D('',#22947,#18283,#18284);
#18175=DIRECTION('axis',(0.,0.,1.));
#18176=DIRECTION('refdir',(1.,0.,0.));
#18177=DIRECTION('center_axis',(0.,0.,1.));
#18178=DIRECTION('ref_axis',(1.,0.,0.));
#18179=DIRECTION('center_axis',(0.,-1.,0.));
#18180=DIRECTION('ref_axis',(0.,0.,-1.));
#18181=DIRECTION('center_axis',(0.,-1.,0.));
#18182=DIRECTION('ref_axis',(0.,0.,-1.));
#18183=DIRECTION('center_axis',(0.,1.,0.));
#18184=DIRECTION('ref_axis',(1.,0.,0.));
#18185=DIRECTION('center_axis',(0.,1.,0.));
#18186=DIRECTION('ref_axis',(1.,0.,0.));
#18187=DIRECTION('center_axis',(0.,1.,0.));
#18188=DIRECTION('ref_axis',(1.,0.,0.));
#18189=DIRECTION('center_axis',(0.,1.,0.));
#18190=DIRECTION('ref_axis',(1.,0.,0.));
#18191=DIRECTION('',(0.,-1.,0.));
#18192=DIRECTION('center_axis',(0.,-1.,0.));
#18193=DIRECTION('ref_axis',(1.,0.,0.));
#18194=DIRECTION('center_axis',(0.,1.,0.));
#18195=DIRECTION('ref_axis',(1.,0.,0.));
#18196=DIRECTION('center_axis',(0.,1.,0.));
#18197=DIRECTION('ref_axis',(1.,0.,0.));
#18198=DIRECTION('center_axis',(0.,1.,0.));
#18199=DIRECTION('ref_axis',(1.,0.,0.));
#18200=DIRECTION('center_axis',(0.,1.,0.));
#18201=DIRECTION('ref_axis',(1.,0.,0.));
#18202=DIRECTION('center_axis',(0.,1.,0.));
#18203=DIRECTION('ref_axis',(1.,0.,0.));
#18204=DIRECTION('center_axis',(0.,1.,0.));
#18205=DIRECTION('ref_axis',(1.,0.,0.));
#18206=DIRECTION('center_axis',(0.,-1.,0.));
#18207=DIRECTION('ref_axis',(1.,0.,0.));
#18208=DIRECTION('center_axis',(0.,-1.,0.));
#18209=DIRECTION('ref_axis',(0.,0.,-1.));
#18210=DIRECTION('center_axis',(6.12323399573677E-17,0.,1.));
#18211=DIRECTION('ref_axis',(1.,0.,0.));
#18212=DIRECTION('center_axis',(0.,-1.,0.));
#18213=DIRECTION('ref_axis',(0.,0.,-1.));
#18214=DIRECTION('center_axis',(0.,1.,0.));
#18215=DIRECTION('ref_axis',(1.,0.,0.));
#18216=DIRECTION('center_axis',(0.,-1.,0.));
#18217=DIRECTION('ref_axis',(1.,0.,0.));
#18218=DIRECTION('center_axis',(0.,-1.,0.));
#18219=DIRECTION('ref_axis',(0.,0.,-1.));
#18220=DIRECTION('center_axis',(0.,0.,1.));
#18221=DIRECTION('ref_axis',(1.,0.,0.));
#18222=DIRECTION('center_axis',(0.,-1.,0.));
#18223=DIRECTION('ref_axis',(0.,0.,-1.));
#18224=DIRECTION('center_axis',(0.,1.,0.));
#18225=DIRECTION('ref_axis',(1.,0.,0.));
#18226=DIRECTION('center_axis',(0.,-1.,0.));
#18227=DIRECTION('ref_axis',(1.,0.,0.));
#18228=DIRECTION('center_axis',(0.,-1.,0.));
#18229=DIRECTION('ref_axis',(0.,0.,-1.));
#18230=DIRECTION('center_axis',(0.,0.,1.));
#18231=DIRECTION('ref_axis',(1.,0.,0.));
#18232=DIRECTION('center_axis',(0.,-1.,0.));
#18233=DIRECTION('ref_axis',(0.,0.,-1.));
#18234=DIRECTION('center_axis',(0.,1.,0.));
#18235=DIRECTION('ref_axis',(1.,0.,0.));
#18236=DIRECTION('center_axis',(0.,-1.,0.));
#18237=DIRECTION('ref_axis',(1.,0.,0.));
#18238=DIRECTION('center_axis',(0.,-1.,0.));
#18239=DIRECTION('ref_axis',(0.,0.,-1.));
#18240=DIRECTION('center_axis',(0.,0.,1.));
#18241=DIRECTION('ref_axis',(1.,0.,0.));
#18242=DIRECTION('center_axis',(0.,-1.,0.));
#18243=DIRECTION('ref_axis',(0.,0.,-1.));
#18244=DIRECTION('center_axis',(0.,1.,0.));
#18245=DIRECTION('ref_axis',(1.,0.,0.));
#18246=DIRECTION('center_axis',(0.,-1.,0.));
#18247=DIRECTION('ref_axis',(1.,0.,0.));
#18248=DIRECTION('center_axis',(0.,-1.,0.));
#18249=DIRECTION('ref_axis',(0.,0.,-1.));
#18250=DIRECTION('center_axis',(6.12323399573676E-17,0.,1.));
#18251=DIRECTION('ref_axis',(1.,0.,0.));
#18252=DIRECTION('center_axis',(0.,-1.,0.));
#18253=DIRECTION('ref_axis',(0.,0.,-1.));
#18254=DIRECTION('center_axis',(0.,1.,0.));
#18255=DIRECTION('ref_axis',(1.,0.,0.));
#18256=DIRECTION('center_axis',(0.,-1.,0.));
#18257=DIRECTION('ref_axis',(1.,0.,0.));
#18258=DIRECTION('center_axis',(0.,-1.,0.));
#18259=DIRECTION('ref_axis',(0.,0.,-1.));
#18260=DIRECTION('center_axis',(0.,0.,1.));
#18261=DIRECTION('ref_axis',(1.,0.,0.));
#18262=DIRECTION('center_axis',(0.,-1.,0.));
#18263=DIRECTION('ref_axis',(0.,0.,-1.));
#18264=DIRECTION('center_axis',(0.,1.,0.));
#18265=DIRECTION('ref_axis',(1.,0.,0.));
#18266=DIRECTION('center_axis',(0.,1.,0.));
#18267=DIRECTION('ref_axis',(1.,0.,0.));
#18268=DIRECTION('',(0.,1.,0.));
#18269=DIRECTION('center_axis',(0.,-1.,0.));
#18270=DIRECTION('ref_axis',(1.,0.,0.));
#18271=DIRECTION('center_axis',(0.,-1.,0.));
#18272=DIRECTION('ref_axis',(1.,0.,0.));
#18273=DIRECTION('center_axis',(0.,1.,0.));
#18274=DIRECTION('ref_axis',(1.,0.,0.));
#18275=DIRECTION('center_axis',(0.,-1.,0.));
#18276=DIRECTION('ref_axis',(0.,0.,-1.));
#18277=DIRECTION('center_axis',(0.,0.,1.));
#18278=DIRECTION('ref_axis',(1.,0.,0.));
#18279=DIRECTION('center_axis',(0.,-1.,0.));
#18280=DIRECTION('ref_axis',(0.,0.,-1.));
#18281=DIRECTION('center_axis',(0.,-1.,0.));
#18282=DIRECTION('ref_axis',(-1.,0.,0.));
#18283=DIRECTION('center_axis',(0.,1.,0.));
#18284=DIRECTION('ref_axis',(1.,0.,0.));
#22500=CARTESIAN_POINT('',(0.,0.,0.));
#22501=CARTESIAN_POINT('Origin',(0.707106781186547,0.,0.707106781186548));
#22502=CARTESIAN_POINT('',(0.504455939115715,-0.04763,0.841298510752802));
#22503=CARTESIAN_POINT('',(0.841298510752802,-0.04763,0.504455939115715));
#22504=CARTESIAN_POINT('Ctrl Pts',(0.504455939115715,-0.04763,0.841298510752802));
#22505=CARTESIAN_POINT('Ctrl Pts',(0.508899795931835,-0.0740444353928835,
0.838633903678357));
#22506=CARTESIAN_POINT('Ctrl Pts',(0.517157748491652,-0.0999305678883309,
0.833661031856294));
#22507=CARTESIAN_POINT('Ctrl Pts',(0.537715343527944,-0.142345102874864,
0.820511285096538));
#22508=CARTESIAN_POINT('Ctrl Pts',(0.548874290046456,-0.159766064500479,
0.813159949759));
#22509=CARTESIAN_POINT('Ctrl Pts',(0.573915184558107,-0.190326085855194,
0.795684265985089));
#22510=CARTESIAN_POINT('Ctrl Pts',(0.587792702767295,-0.203463743702801,
0.78555112003688));
#22511=CARTESIAN_POINT('Ctrl Pts',(0.615966552324775,-0.224161999508995,
0.763642258217233));
#22512=CARTESIAN_POINT('Ctrl Pts',(0.631684198665438,-0.232861760990032,
0.750785745543687));
#22513=CARTESIAN_POINT('Ctrl Pts',(0.663382628119203,-0.244251601209411,
0.722929908501543));
#22514=CARTESIAN_POINT('Ctrl Pts',(0.679352081686668,-0.246942143572133,
0.707917883896095));
#22515=CARTESIAN_POINT('Ctrl Pts',(0.707917883896095,-0.246942143572133,
0.679352081686668));
#22516=CARTESIAN_POINT('Ctrl Pts',(0.722929908501543,-0.244251601209411,
0.663382628119203));
#22517=CARTESIAN_POINT('Ctrl Pts',(0.750785745543687,-0.232861760990032,
0.631684198665439));
#22518=CARTESIAN_POINT('Ctrl Pts',(0.763642258217232,-0.224161999508995,
0.615966552324775));
#22519=CARTESIAN_POINT('Ctrl Pts',(0.78555112003688,-0.203463743702801,
0.587792702767295));
#22520=CARTESIAN_POINT('Ctrl Pts',(0.795684265985088,-0.190326085855194,
0.573915184558108));
#22521=CARTESIAN_POINT('Ctrl Pts',(0.813159949759,-0.15976606450048,0.548874290046456));
#22522=CARTESIAN_POINT('Ctrl Pts',(0.820511285096538,-0.142345102874864,
0.537715343527944));
#22523=CARTESIAN_POINT('Ctrl Pts',(0.833661031856294,-0.099930567888331,
0.517157748491653));
#22524=CARTESIAN_POINT('Ctrl Pts',(0.838633903678357,-0.0740444353928835,
0.508899795931835));
#22525=CARTESIAN_POINT('Ctrl Pts',(0.841298510752801,-0.0476299999999999,
0.504455939115715));
#22526=CARTESIAN_POINT('',(0.528110872004958,-0.04763,0.871530771444223));
#22527=CARTESIAN_POINT('Origin',(0.707106781186547,-0.04763,0.707106781186548));
#22528=CARTESIAN_POINT('',(0.871530771444223,-0.04763,0.528110872004959));
#22529=CARTESIAN_POINT('Ctrl Pts',(0.871530771444223,-0.0476300000000001,
0.528110872004958));
#22530=CARTESIAN_POINT('Ctrl Pts',(0.87014664509073,-0.0609922781173483,
0.530395067942936));
#22531=CARTESIAN_POINT('Ctrl Pts',(0.868149331745851,-0.0742967091364493,
0.533674141594226));
#22532=CARTESIAN_POINT('Ctrl Pts',(0.85981294420286,-0.115492077056649,
0.54708917182331));
#22533=CARTESIAN_POINT('Ctrl Pts',(0.850993704737257,-0.141695629206859,
0.560922177770136));
#22534=CARTESIAN_POINT('Ctrl Pts',(0.830754510485543,-0.181890537957859,
0.590422647829571));
#22535=CARTESIAN_POINT('Ctrl Pts',(0.816896541396381,-0.201072148666545,
0.609616703125488));
#22536=CARTESIAN_POINT('Ctrl Pts',(0.792310597819928,-0.223955109275652,
0.641117951819998));
#22537=CARTESIAN_POINT('Ctrl Pts',(0.779109323683612,-0.232742381310829,
0.657208095763053));
#22538=CARTESIAN_POINT('Ctrl Pts',(0.750552691816206,-0.244234834628584,
0.68964083160521));
#22539=CARTESIAN_POINT('Ctrl Pts',(0.735185187071673,-0.246942143572133,
0.705971972091755));
#22540=CARTESIAN_POINT('Ctrl Pts',(0.705971972091754,-0.246942143572133,
0.735185187071673));
#22541=CARTESIAN_POINT('Ctrl Pts',(0.689640831605209,-0.244234834628584,
0.750552691816206));
#22542=CARTESIAN_POINT('Ctrl Pts',(0.657208095763052,-0.232742381310829,
0.779109323683612));
#22543=CARTESIAN_POINT('Ctrl Pts',(0.641117951819998,-0.223955109275652,
0.792310597819928));
#22544=CARTESIAN_POINT('Ctrl Pts',(0.609616703125487,-0.201072148666545,
0.816896541396382));
#22545=CARTESIAN_POINT('Ctrl Pts',(0.590422647829571,-0.181890537957858,
0.830754510485544));
#22546=CARTESIAN_POINT('Ctrl Pts',(0.560922177770135,-0.141695629206858,
0.850993704737257));
#22547=CARTESIAN_POINT('Ctrl Pts',(0.547089171823309,-0.115492077056649,
0.859812944202861));
#22548=CARTESIAN_POINT('Ctrl Pts',(0.533674141594226,-0.0742967091364491,
0.868149331745852));
#22549=CARTESIAN_POINT('Ctrl Pts',(0.530395067942936,-0.0609922781173483,
0.870146645090731));
#22550=CARTESIAN_POINT('Ctrl Pts',(0.528110872004958,-0.0476300000000001,
0.871530771444223));
#22551=CARTESIAN_POINT('Origin',(0.707106781186547,-0.04763,0.707106781186548));
#22552=CARTESIAN_POINT('Origin',(0.,-0.166705,0.));
#22553=CARTESIAN_POINT('',(0.242834539687906,-0.04763,0.989696097314));
#22554=CARTESIAN_POINT('Origin',(0.,-0.04763,0.));
#22555=CARTESIAN_POINT('',(-0.242834539687907,-0.04763,0.989696097314));
#22556=CARTESIAN_POINT('Ctrl Pts',(0.242834539687906,-0.04763,0.989696097314));
#22557=CARTESIAN_POINT('Ctrl Pts',(0.24024064412003,-0.0609922781173483,
0.990332542620729));
#22558=CARTESIAN_POINT('Ctrl Pts',(0.236509675094874,-0.0742967091364492,
0.991238884025248));
#22559=CARTESIAN_POINT('Ctrl Pts',(0.221129100087819,-0.115492077056649,
0.994830026707808));
#22560=CARTESIAN_POINT('Ctrl Pts',(0.205111543747588,-0.141695629206859,
0.998375294985966));
#22561=CARTESIAN_POINT('Ctrl Pts',(0.169940289819232,-0.181890537957859,
1.00492400591205));
#22562=CARTESIAN_POINT('Ctrl Pts',(0.1465689792446,-0.201072148666545,1.00869718865384));
#22563=CARTESIAN_POINT('Ctrl Pts',(0.106909345252087,-0.223955109275652,
1.01358704779679));
#22564=CARTESIAN_POINT('Ctrl Pts',(0.0861971848975941,-0.232742381310829,
1.0156297872271));
#22565=CARTESIAN_POINT('Ctrl Pts',(0.0430711894098822,-0.244234834628584,
1.01837060663223));
#22566=CARTESIAN_POINT('Ctrl Pts',(0.0206568624125605,-0.246942143572133,
1.019052));
#22567=CARTESIAN_POINT('Ctrl Pts',(-0.0206568624125608,-0.246942143572133,
1.019052));
#22568=CARTESIAN_POINT('Ctrl Pts',(-0.0430711894098825,-0.244234834628584,
1.01837060663223));
#22569=CARTESIAN_POINT('Ctrl Pts',(-0.0861971848975943,-0.232742381310829,
1.0156297872271));
#22570=CARTESIAN_POINT('Ctrl Pts',(-0.106909345252088,-0.223955109275652,
1.01358704779679));
#22571=CARTESIAN_POINT('Ctrl Pts',(-0.1465689792446,-0.201072148666545,
1.00869718865384));
#22572=CARTESIAN_POINT('Ctrl Pts',(-0.169940289819232,-0.181890537957859,
1.00492400591205));
#22573=CARTESIAN_POINT('Ctrl Pts',(-0.205111543747588,-0.141695629206859,
0.998375294985966));
#22574=CARTESIAN_POINT('Ctrl Pts',(-0.221129100087819,-0.115492077056649,
0.994830026707808));
#22575=CARTESIAN_POINT('Ctrl Pts',(-0.236509675094875,-0.0742967091364493,
0.991238884025248));
#22576=CARTESIAN_POINT('Ctrl Pts',(-0.24024064412003,-0.0609922781173483,
0.990332542620729));
#22577=CARTESIAN_POINT('Ctrl Pts',(-0.242834539687907,-0.04763,0.989696097314));
#22578=CARTESIAN_POINT('',(-0.528110872004959,-0.04763,0.871530771444223));
#22579=CARTESIAN_POINT('Origin',(0.,-0.04763,0.));
#22580=CARTESIAN_POINT('',(-0.871530771444223,-0.04763,0.528110872004958));
#22581=CARTESIAN_POINT('Ctrl Pts',(-0.528110872004958,-0.0476300000000001,
0.871530771444223));
#22582=CARTESIAN_POINT('Ctrl Pts',(-0.530395067942936,-0.0609922781173484,
0.87014664509073));
#22583=CARTESIAN_POINT('Ctrl Pts',(-0.533674141594226,-0.0742967091364493,
0.868149331745851));
#22584=CARTESIAN_POINT('Ctrl Pts',(-0.54708917182331,-0.115492077056649,
0.85981294420286));
#22585=CARTESIAN_POINT('Ctrl Pts',(-0.560922177770136,-0.141695629206859,
0.850993704737257));
#22586=CARTESIAN_POINT('Ctrl Pts',(-0.590422647829571,-0.181890537957859,
0.830754510485543));
#22587=CARTESIAN_POINT('Ctrl Pts',(-0.609616703125488,-0.201072148666545,
0.816896541396381));
#22588=CARTESIAN_POINT('Ctrl Pts',(-0.641117951819998,-0.223955109275652,
0.792310597819928));
#22589=CARTESIAN_POINT('Ctrl Pts',(-0.657208095763053,-0.232742381310829,
0.779109323683611));
#22590=CARTESIAN_POINT('Ctrl Pts',(-0.68964083160521,-0.244234834628584,
0.750552691816205));
#22591=CARTESIAN_POINT('Ctrl Pts',(-0.705971972091755,-0.246942143572133,
0.735185187071673));
#22592=CARTESIAN_POINT('Ctrl Pts',(-0.735185187071673,-0.246942143572133,
0.705971972091754));
#22593=CARTESIAN_POINT('Ctrl Pts',(-0.750552691816206,-0.244234834628584,
0.689640831605209));
#22594=CARTESIAN_POINT('Ctrl Pts',(-0.779109323683612,-0.232742381310829,
0.657208095763052));
#22595=CARTESIAN_POINT('Ctrl Pts',(-0.792310597819928,-0.223955109275652,
0.641117951819998));
#22596=CARTESIAN_POINT('Ctrl Pts',(-0.816896541396382,-0.201072148666545,
0.609616703125487));
#22597=CARTESIAN_POINT('Ctrl Pts',(-0.830754510485544,-0.181890537957858,
0.590422647829571));
#22598=CARTESIAN_POINT('Ctrl Pts',(-0.850993704737257,-0.141695629206858,
0.560922177770135));
#22599=CARTESIAN_POINT('Ctrl Pts',(-0.859812944202861,-0.115492077056649,
0.547089171823309));
#22600=CARTESIAN_POINT('Ctrl Pts',(-0.868149331745852,-0.0742967091364491,
0.533674141594226));
#22601=CARTESIAN_POINT('Ctrl Pts',(-0.870146645090731,-0.0609922781173483,
0.530395067942936));
#22602=CARTESIAN_POINT('Ctrl Pts',(-0.871530771444223,-0.04763,0.528110872004958));
#22603=CARTESIAN_POINT('',(-0.989696097314,-0.04763,0.242834539687906));
#22604=CARTESIAN_POINT('Origin',(0.,-0.04763,0.));
#22605=CARTESIAN_POINT('',(-1.019052,-0.246942143572133,1.248489836334E-16));
#22606=CARTESIAN_POINT('Ctrl Pts',(-0.989696097314,-0.04763,0.242834539687906));
#22607=CARTESIAN_POINT('Ctrl Pts',(-0.990332542620729,-0.0609922781173483,
0.24024064412003));
#22608=CARTESIAN_POINT('Ctrl Pts',(-0.991238884025248,-0.0742967091364492,
0.236509675094874));
#22609=CARTESIAN_POINT('Ctrl Pts',(-0.994830026707808,-0.115492077056649,
0.221129100087819));
#22610=CARTESIAN_POINT('Ctrl Pts',(-0.998375294985966,-0.141695629206859,
0.205111543747588));
#22611=CARTESIAN_POINT('Ctrl Pts',(-1.00492400591205,-0.181890537957859,
0.169940289819232));
#22612=CARTESIAN_POINT('Ctrl Pts',(-1.00869718865384,-0.201072148666545,
0.1465689792446));
#22613=CARTESIAN_POINT('Ctrl Pts',(-1.01358704779679,-0.223955109275652,
0.106909345252088));
#22614=CARTESIAN_POINT('Ctrl Pts',(-1.0156297872271,-0.232742381310829,
0.0861971848975944));
#22615=CARTESIAN_POINT('Ctrl Pts',(-1.01837060663223,-0.244234834628584,
0.0430711894098825));
#22616=CARTESIAN_POINT('Ctrl Pts',(-1.019052,-0.246942143572133,0.0206568624125608));
#22617=CARTESIAN_POINT('Ctrl Pts',(-1.019052,-0.246942143572133,1.2490009027033E-16));
#22618=CARTESIAN_POINT('',(-1.019052,-0.28578,1.24797876996471E-16));
#22619=CARTESIAN_POINT('',(-1.019052,-0.166705,1.24797876996471E-16));
#22620=CARTESIAN_POINT('Origin',(0.,-0.28578,0.));
#22621=CARTESIAN_POINT('',(-0.989696097314,-0.04763,-0.242834539687906));
#22622=CARTESIAN_POINT('Ctrl Pts',(-1.019052,-0.246942143572133,1.2490009027033E-16));
#22623=CARTESIAN_POINT('Ctrl Pts',(-1.019052,-0.246942143572133,-0.0206568624125605));
#22624=CARTESIAN_POINT('Ctrl Pts',(-1.01837060663223,-0.244234834628584,
-0.0430711894098822));
#22625=CARTESIAN_POINT('Ctrl Pts',(-1.0156297872271,-0.232742381310829,
-0.0861971848975941));
#22626=CARTESIAN_POINT('Ctrl Pts',(-1.01358704779679,-0.223955109275652,
-0.106909345252087));
#22627=CARTESIAN_POINT('Ctrl Pts',(-1.00869718865384,-0.201072148666546,
-0.1465689792446));
#22628=CARTESIAN_POINT('Ctrl Pts',(-1.00492400591205,-0.181890537957859,
-0.169940289819232));
#22629=CARTESIAN_POINT('Ctrl Pts',(-0.998375294985966,-0.141695629206859,
-0.205111543747588));
#22630=CARTESIAN_POINT('Ctrl Pts',(-0.994830026707808,-0.11549207705665,
-0.221129100087819));
#22631=CARTESIAN_POINT('Ctrl Pts',(-0.991238884025248,-0.0742967091364495,
-0.236509675094874));
#22632=CARTESIAN_POINT('Ctrl Pts',(-0.990332542620729,-0.0609922781173484,
-0.24024064412003));
#22633=CARTESIAN_POINT('Ctrl Pts',(-0.989696097314,-0.0476300000000001,
-0.242834539687907));
#22634=CARTESIAN_POINT('',(-0.871530771444223,-0.04763,-0.528110872004958));
#22635=CARTESIAN_POINT('Origin',(0.,-0.04763,0.));
#22636=CARTESIAN_POINT('',(-0.528110872004958,-0.04763,-0.871530771444223));
#22637=CARTESIAN_POINT('Ctrl Pts',(-0.871530771444223,-0.0476300000000001,
-0.528110872004958));
#22638=CARTESIAN_POINT('Ctrl Pts',(-0.87014664509073,-0.0609922781173484,
-0.530395067942936));
#22639=CARTESIAN_POINT('Ctrl Pts',(-0.868149331745851,-0.0742967091364494,
-0.533674141594226));
#22640=CARTESIAN_POINT('Ctrl Pts',(-0.85981294420286,-0.115492077056649,
-0.54708917182331));
#22641=CARTESIAN_POINT('Ctrl Pts',(-0.850993704737257,-0.141695629206859,
-0.560922177770136));
#22642=CARTESIAN_POINT('Ctrl Pts',(-0.830754510485543,-0.181890537957859,
-0.590422647829571));
#22643=CARTESIAN_POINT('Ctrl Pts',(-0.816896541396381,-0.201072148666546,
-0.609616703125488));
#22644=CARTESIAN_POINT('Ctrl Pts',(-0.792310597819928,-0.223955109275652,
-0.641117951819999));
#22645=CARTESIAN_POINT('Ctrl Pts',(-0.779109323683611,-0.232742381310829,
-0.657208095763053));
#22646=CARTESIAN_POINT('Ctrl Pts',(-0.750552691816205,-0.244234834628584,
-0.68964083160521));
#22647=CARTESIAN_POINT('Ctrl Pts',(-0.735185187071673,-0.246942143572133,
-0.705971972091755));
#22648=CARTESIAN_POINT('Ctrl Pts',(-0.705971972091754,-0.246942143572133,
-0.735185187071673));
#22649=CARTESIAN_POINT('Ctrl Pts',(-0.68964083160521,-0.244234834628584,
-0.750552691816206));
#22650=CARTESIAN_POINT('Ctrl Pts',(-0.657208095763052,-0.232742381310829,
-0.779109323683612));
#22651=CARTESIAN_POINT('Ctrl Pts',(-0.641117951819998,-0.223955109275652,
-0.792310597819928));
#22652=CARTESIAN_POINT('Ctrl Pts',(-0.609616703125488,-0.201072148666545,
-0.816896541396381));
#22653=CARTESIAN_POINT('Ctrl Pts',(-0.590422647829571,-0.181890537957859,
-0.830754510485543));
#22654=CARTESIAN_POINT('Ctrl Pts',(-0.560922177770136,-0.141695629206859,
-0.850993704737257));
#22655=CARTESIAN_POINT('Ctrl Pts',(-0.54708917182331,-0.115492077056649,
-0.85981294420286));
#22656=CARTESIAN_POINT('Ctrl Pts',(-0.533674141594226,-0.0742967091364494,
-0.868149331745852));
#22657=CARTESIAN_POINT('Ctrl Pts',(-0.530395067942936,-0.0609922781173484,
-0.870146645090731));
#22658=CARTESIAN_POINT('Ctrl Pts',(-0.528110872004958,-0.0476300000000001,
-0.871530771444223));
#22659=CARTESIAN_POINT('',(-0.242834539687906,-0.04763,-0.989696097314));
#22660=CARTESIAN_POINT('Origin',(0.,-0.04763,0.));
#22661=CARTESIAN_POINT('',(0.242834539687906,-0.04763,-0.989696097314));
#22662=CARTESIAN_POINT('Ctrl Pts',(-0.242834539687907,-0.04763,-0.989696097314));
#22663=CARTESIAN_POINT('Ctrl Pts',(-0.24024064412003,-0.0609922781173483,
-0.990332542620729));
#22664=CARTESIAN_POINT('Ctrl Pts',(-0.236509675094874,-0.0742967091364493,
-0.991238884025248));
#22665=CARTESIAN_POINT('Ctrl Pts',(-0.221129100087819,-0.115492077056649,
-0.994830026707808));
#22666=CARTESIAN_POINT('Ctrl Pts',(-0.205111543747588,-0.141695629206859,
-0.998375294985966));
#22667=CARTESIAN_POINT('Ctrl Pts',(-0.169940289819232,-0.181890537957859,
-1.00492400591205));
#22668=CARTESIAN_POINT('Ctrl Pts',(-0.1465689792446,-0.201072148666545,
-1.00869718865384));
#22669=CARTESIAN_POINT('Ctrl Pts',(-0.106909345252087,-0.223955109275652,
-1.01358704779679));
#22670=CARTESIAN_POINT('Ctrl Pts',(-0.0861971848975942,-0.232742381310829,
-1.0156297872271));
#22671=CARTESIAN_POINT('Ctrl Pts',(-0.0430711894098823,-0.244234834628584,
-1.01837060663223));
#22672=CARTESIAN_POINT('Ctrl Pts',(-0.0206568624125606,-0.246942143572133,
-1.019052));
#22673=CARTESIAN_POINT('Ctrl Pts',(0.0206568624125607,-0.246942143572133,
-1.019052));
#22674=CARTESIAN_POINT('Ctrl Pts',(0.0430711894098824,-0.244234834628584,
-1.01837060663223));
#22675=CARTESIAN_POINT('Ctrl Pts',(0.0861971848975943,-0.232742381310829,
-1.0156297872271));
#22676=CARTESIAN_POINT('Ctrl Pts',(0.106909345252088,-0.223955109275652,
-1.01358704779679));
#22677=CARTESIAN_POINT('Ctrl Pts',(0.1465689792446,-0.201072148666545,-1.00869718865384));
#22678=CARTESIAN_POINT('Ctrl Pts',(0.169940289819232,-0.181890537957859,
-1.00492400591205));
#22679=CARTESIAN_POINT('Ctrl Pts',(0.205111543747588,-0.141695629206859,
-0.998375294985966));
#22680=CARTESIAN_POINT('Ctrl Pts',(0.221129100087819,-0.115492077056649,
-0.994830026707808));
#22681=CARTESIAN_POINT('Ctrl Pts',(0.236509675094874,-0.0742967091364493,
-0.991238884025248));
#22682=CARTESIAN_POINT('Ctrl Pts',(0.24024064412003,-0.0609922781173484,
-0.990332542620729));
#22683=CARTESIAN_POINT('Ctrl Pts',(0.242834539687907,-0.04763,-0.989696097314));
#22684=CARTESIAN_POINT('',(0.528110872004958,-0.04763,-0.871530771444223));
#22685=CARTESIAN_POINT('Origin',(0.,-0.04763,0.));
#22686=CARTESIAN_POINT('',(0.871530771444223,-0.04763,-0.528110872004958));
#22687=CARTESIAN_POINT('Ctrl Pts',(0.528110872004958,-0.0476300000000001,
-0.871530771444223));
#22688=CARTESIAN_POINT('Ctrl Pts',(0.530395067942936,-0.0609922781173484,
-0.870146645090731));
#22689=CARTESIAN_POINT('Ctrl Pts',(0.533674141594226,-0.0742967091364493,
-0.868149331745851));
#22690=CARTESIAN_POINT('Ctrl Pts',(0.54708917182331,-0.115492077056649,
-0.85981294420286));
#22691=CARTESIAN_POINT('Ctrl Pts',(0.560922177770136,-0.141695629206859,
-0.850993704737257));
#22692=CARTESIAN_POINT('Ctrl Pts',(0.590422647829571,-0.181890537957859,
-0.830754510485543));
#22693=CARTESIAN_POINT('Ctrl Pts',(0.609616703125488,-0.201072148666545,
-0.816896541396381));
#22694=CARTESIAN_POINT('Ctrl Pts',(0.641117951819998,-0.223955109275652,
-0.792310597819928));
#22695=CARTESIAN_POINT('Ctrl Pts',(0.657208095763053,-0.232742381310829,
-0.779109323683612));
#22696=CARTESIAN_POINT('Ctrl Pts',(0.68964083160521,-0.244234834628584,
-0.750552691816206));
#22697=CARTESIAN_POINT('Ctrl Pts',(0.705971972091755,-0.246942143572133,
-0.735185187071673));
#22698=CARTESIAN_POINT('Ctrl Pts',(0.735185187071673,-0.246942143572133,
-0.705971972091754));
#22699=CARTESIAN_POINT('Ctrl Pts',(0.750552691816206,-0.244234834628584,
-0.68964083160521));
#22700=CARTESIAN_POINT('Ctrl Pts',(0.779109323683612,-0.232742381310829,
-0.657208095763053));
#22701=CARTESIAN_POINT('Ctrl Pts',(0.792310597819928,-0.223955109275652,
-0.641117951819998));
#22702=CARTESIAN_POINT('Ctrl Pts',(0.816896541396381,-0.201072148666545,
-0.609616703125488));
#22703=CARTESIAN_POINT('Ctrl Pts',(0.830754510485543,-0.181890537957859,
-0.590422647829571));
#22704=CARTESIAN_POINT('Ctrl Pts',(0.850993704737257,-0.141695629206859,
-0.560922177770136));
#22705=CARTESIAN_POINT('Ctrl Pts',(0.85981294420286,-0.115492077056649,
-0.54708917182331));
#22706=CARTESIAN_POINT('Ctrl Pts',(0.868149331745851,-0.0742967091364493,
-0.533674141594226));
#22707=CARTESIAN_POINT('Ctrl Pts',(0.870146645090731,-0.0609922781173484,
-0.530395067942936));
#22708=CARTESIAN_POINT('Ctrl Pts',(0.871530771444223,-0.0476300000000001,
-0.528110872004958));
#22709=CARTESIAN_POINT('',(0.989696097314,-0.04763,-0.242834539687906));
#22710=CARTESIAN_POINT('Origin',(0.,-0.04763,0.));
#22711=CARTESIAN_POINT('',(0.989696097314,-0.04763,0.242834539687906));
#22712=CARTESIAN_POINT('Ctrl Pts',(0.989696097314,-0.04763,-0.242834539687907));
#22713=CARTESIAN_POINT('Ctrl Pts',(0.990332542620729,-0.0609922781173483,
-0.24024064412003));
#22714=CARTESIAN_POINT('Ctrl Pts',(0.991238884025248,-0.0742967091364493,
-0.236509675094874));
#22715=CARTESIAN_POINT('Ctrl Pts',(0.994830026707808,-0.115492077056649,
-0.221129100087819));
#22716=CARTESIAN_POINT('Ctrl Pts',(0.998375294985966,-0.141695629206859,
-0.205111543747588));
#22717=CARTESIAN_POINT('Ctrl Pts',(1.00492400591205,-0.181890537957859,
-0.169940289819232));
#22718=CARTESIAN_POINT('Ctrl Pts',(1.00869718865384,-0.201072148666545,
-0.1465689792446));
#22719=CARTESIAN_POINT('Ctrl Pts',(1.01358704779679,-0.223955109275652,
-0.106909345252087));
#22720=CARTESIAN_POINT('Ctrl Pts',(1.0156297872271,-0.232742381310829,-0.0861971848975942));
#22721=CARTESIAN_POINT('Ctrl Pts',(1.01837060663223,-0.244234834628584,
-0.0430711894098823));
#22722=CARTESIAN_POINT('Ctrl Pts',(1.019052,-0.246942143572133,-0.0206568624125607));
#22723=CARTESIAN_POINT('Ctrl Pts',(1.019052,-0.246942143572133,0.0206568624125607));
#22724=CARTESIAN_POINT('Ctrl Pts',(1.01837060663223,-0.244234834628584,
0.0430711894098823));
#22725=CARTESIAN_POINT('Ctrl Pts',(1.0156297872271,-0.232742381310829,0.0861971848975942));
#22726=CARTESIAN_POINT('Ctrl Pts',(1.01358704779679,-0.223955109275652,
0.106909345252087));
#22727=CARTESIAN_POINT('Ctrl Pts',(1.00869718865384,-0.201072148666545,
0.1465689792446));
#22728=CARTESIAN_POINT('Ctrl Pts',(1.00492400591205,-0.181890537957859,
0.169940289819232));
#22729=CARTESIAN_POINT('Ctrl Pts',(0.998375294985966,-0.141695629206859,
0.205111543747588));
#22730=CARTESIAN_POINT('Ctrl Pts',(0.994830026707808,-0.115492077056649,
0.221129100087819));
#22731=CARTESIAN_POINT('Ctrl Pts',(0.991238884025248,-0.0742967091364492,
0.236509675094874));
#22732=CARTESIAN_POINT('Ctrl Pts',(0.990332542620729,-0.0609922781173483,
0.24024064412003));
#22733=CARTESIAN_POINT('Ctrl Pts',(0.989696097314,-0.04763,0.242834539687907));
#22734=CARTESIAN_POINT('Origin',(0.,-0.04763,0.));
#22735=CARTESIAN_POINT('Origin',(0.,-0.04763,0.));
#22736=CARTESIAN_POINT('',(0.238183666596899,-0.04763,0.951592097314));
#22737=CARTESIAN_POINT('Origin',(0.,-0.04763,0.));
#22738=CARTESIAN_POINT('Origin',(-1.94289029309402E-16,-0.04763,1.));
#22739=CARTESIAN_POINT('Origin',(-1.94289029309402E-16,0.,1.));
#22740=CARTESIAN_POINT('',(-0.2381836665969,-0.04763,0.951592097314));
#22741=CARTESIAN_POINT('Ctrl Pts',(-0.238183666596899,-0.0476299999999999,
0.951592097314));
#22742=CARTESIAN_POINT('Ctrl Pts',(-0.233157223576062,-0.0740444353928835,
0.952850216871763));
#22743=CARTESIAN_POINT('Ctrl Pts',(-0.223801617934946,-0.0999305678883309,
0.955173119738174));
#22744=CARTESIAN_POINT('Ctrl Pts',(-0.199966927975188,-0.142345102874864,
0.960411259488514));
#22745=CARTESIAN_POINT('Ctrl Pts',(-0.1868781821531,-0.159766064500479,
0.963103647174702));
#22746=CARTESIAN_POINT('Ctrl Pts',(-0.15681442133453,-0.190326085855194,
0.968453058988463));
#22747=CARTESIAN_POINT('Ctrl Pts',(-0.139836317888043,-0.203463743702801,
0.971100730005489));
#22748=CARTESIAN_POINT('Ctrl Pts',(-0.104422493053067,-0.224161999508995,
0.975530745318961));
#22749=CARTESIAN_POINT('Ctrl Pts',(-0.0842175114474176,-0.232861760990032,
0.977553872336861));
#22750=CARTESIAN_POINT('Ctrl Pts',(-0.0421062857595701,-0.244251601209411,
0.980270995488453));
#22751=CARTESIAN_POINT('Ctrl Pts',(-0.0201990724523197,-0.246942143572133,
0.980948));
#22752=CARTESIAN_POINT('Ctrl Pts',(0.020199072452319,-0.246942143572133,
0.980948));
#22753=CARTESIAN_POINT('Ctrl Pts',(0.0421062857595694,-0.244251601209411,
0.980270995488454));
#22754=CARTESIAN_POINT('Ctrl Pts',(0.0842175114474169,-0.232861760990032,
0.977553872336861));
#22755=CARTESIAN_POINT('Ctrl Pts',(0.104422493053067,-0.224161999508995,
0.975530745318961));
#22756=CARTESIAN_POINT('Ctrl Pts',(0.139836317888042,-0.203463743702801,
0.971100730005489));
#22757=CARTESIAN_POINT('Ctrl Pts',(0.15681442133453,-0.190326085855194,
0.968453058988463));
#22758=CARTESIAN_POINT('Ctrl Pts',(0.1868781821531,-0.15976606450048,0.963103647174702));
#22759=CARTESIAN_POINT('Ctrl Pts',(0.199966927975188,-0.142345102874864,
0.960411259488514));
#22760=CARTESIAN_POINT('Ctrl Pts',(0.223801617934945,-0.0999305678883309,
0.955173119738174));
#22761=CARTESIAN_POINT('Ctrl Pts',(0.233157223576061,-0.0740444353928835,
0.952850216871763));
#22762=CARTESIAN_POINT('Ctrl Pts',(0.238183666596899,-0.0476299999999999,
0.951592097314));
#22763=CARTESIAN_POINT('Origin',(-1.94289029309402E-16,-0.04763,1.));
#22764=CARTESIAN_POINT('Origin',(0.,-0.04763,0.));
#22765=CARTESIAN_POINT('',(-0.504455939115715,-0.04763,0.841298510752802));
#22766=CARTESIAN_POINT('Origin',(0.,-0.04763,0.));
#22767=CARTESIAN_POINT('Origin',(-0.707106781186548,-0.04763,0.707106781186547));
#22768=CARTESIAN_POINT('Origin',(-0.707106781186548,0.,0.707106781186547));
#22769=CARTESIAN_POINT('',(-0.841298510752802,-0.04763,0.504455939115715));
#22770=CARTESIAN_POINT('Ctrl Pts',(-0.841298510752802,-0.04763,0.504455939115715));
#22771=CARTESIAN_POINT('Ctrl Pts',(-0.838633903678357,-0.0740444353928835,
0.508899795931835));
#22772=CARTESIAN_POINT('Ctrl Pts',(-0.833661031856294,-0.0999305678883309,
0.517157748491652));
#22773=CARTESIAN_POINT('Ctrl Pts',(-0.820511285096538,-0.142345102874864,
0.537715343527944));
#22774=CARTESIAN_POINT('Ctrl Pts',(-0.813159949759,-0.159766064500479,0.548874290046456));
#22775=CARTESIAN_POINT('Ctrl Pts',(-0.795684265985089,-0.190326085855194,
0.573915184558107));
#22776=CARTESIAN_POINT('Ctrl Pts',(-0.78555112003688,-0.203463743702801,
0.587792702767295));
#22777=CARTESIAN_POINT('Ctrl Pts',(-0.763642258217233,-0.224161999508995,
0.615966552324775));
#22778=CARTESIAN_POINT('Ctrl Pts',(-0.750785745543687,-0.232861760990032,
0.631684198665438));
#22779=CARTESIAN_POINT('Ctrl Pts',(-0.722929908501543,-0.244251601209411,
0.663382628119203));
#22780=CARTESIAN_POINT('Ctrl Pts',(-0.707917883896095,-0.246942143572133,
0.679352081686668));
#22781=CARTESIAN_POINT('Ctrl Pts',(-0.679352081686668,-0.246942143572133,
0.707917883896095));
#22782=CARTESIAN_POINT('Ctrl Pts',(-0.663382628119203,-0.244251601209411,
0.722929908501544));
#22783=CARTESIAN_POINT('Ctrl Pts',(-0.631684198665438,-0.232861760990031,
0.750785745543687));
#22784=CARTESIAN_POINT('Ctrl Pts',(-0.615966552324775,-0.224161999508995,
0.763642258217233));
#22785=CARTESIAN_POINT('Ctrl Pts',(-0.587792702767295,-0.203463743702801,
0.78555112003688));
#22786=CARTESIAN_POINT('Ctrl Pts',(-0.573915184558107,-0.190326085855194,
0.795684265985088));
#22787=CARTESIAN_POINT('Ctrl Pts',(-0.548874290046456,-0.159766064500479,
0.813159949759));
#22788=CARTESIAN_POINT('Ctrl Pts',(-0.537715343527944,-0.142345102874864,
0.820511285096538));
#22789=CARTESIAN_POINT('Ctrl Pts',(-0.517157748491652,-0.0999305678883309,
0.833661031856294));
#22790=CARTESIAN_POINT('Ctrl Pts',(-0.508899795931835,-0.0740444353928835,
0.838633903678357));
#22791=CARTESIAN_POINT('Ctrl Pts',(-0.504455939115716,-0.04763,0.841298510752801));
#22792=CARTESIAN_POINT('Origin',(-0.707106781186548,-0.04763,0.707106781186547));
#22793=CARTESIAN_POINT('Origin',(0.,-0.04763,0.));
#22794=CARTESIAN_POINT('',(-0.951592097314,-0.04763,0.238183666596899));
#22795=CARTESIAN_POINT('Origin',(0.,-0.04763,0.));
#22796=CARTESIAN_POINT('Origin',(-1.,-0.04763,-1.11022302462516E-16));
#22797=CARTESIAN_POINT('Origin',(-1.,0.,-1.11022302462516E-16));
#22798=CARTESIAN_POINT('',(-0.951592097314,-0.04763,-0.2381836665969));
#22799=CARTESIAN_POINT('',(-0.980948,-0.246942143572133,1.08514323328844E-18));
#22800=CARTESIAN_POINT('Ctrl Pts',(-0.951592097314,-0.04763,-0.238183666596899));
#22801=CARTESIAN_POINT('Ctrl Pts',(-0.952850216871763,-0.0740444353928835,
-0.233157223576062));
#22802=CARTESIAN_POINT('Ctrl Pts',(-0.955173119738174,-0.0999305678883309,
-0.223801617934946));
#22803=CARTESIAN_POINT('Ctrl Pts',(-0.960411259488514,-0.142345102874864,
-0.199966927975188));
#22804=CARTESIAN_POINT('Ctrl Pts',(-0.963103647174702,-0.159766064500479,
-0.1868781821531));
#22805=CARTESIAN_POINT('Ctrl Pts',(-0.968453058988463,-0.190326085855194,
-0.15681442133453));
#22806=CARTESIAN_POINT('Ctrl Pts',(-0.971100730005489,-0.203463743702801,
-0.139836317888043));
#22807=CARTESIAN_POINT('Ctrl Pts',(-0.975530745318961,-0.224161999508995,
-0.104422493053067));
#22808=CARTESIAN_POINT('Ctrl Pts',(-0.977553872336861,-0.232861760990032,
-0.0842175114474175));
#22809=CARTESIAN_POINT('Ctrl Pts',(-0.980270995488453,-0.244251601209411,
-0.0421062857595699));
#22810=CARTESIAN_POINT('Ctrl Pts',(-0.980948,-0.246942143572133,-0.0201990724523195));
#22811=CARTESIAN_POINT('Ctrl Pts',(-0.980948,-0.246942143572133,-1.17961196366423E-16));
#22812=CARTESIAN_POINT('Origin',(-1.,-0.04763,-1.11022302462516E-16));
#22813=CARTESIAN_POINT('Ctrl Pts',(-0.980948,-0.246942143572133,-1.17961196366423E-16));
#22814=CARTESIAN_POINT('Ctrl Pts',(-0.980948,-0.246942143572133,0.0201990724523192));
#22815=CARTESIAN_POINT('Ctrl Pts',(-0.980270995488453,-0.244251601209411,
0.0421062857595695));
#22816=CARTESIAN_POINT('Ctrl Pts',(-0.977553872336861,-0.232861760990032,
0.0842175114474169));
#22817=CARTESIAN_POINT('Ctrl Pts',(-0.975530745318961,-0.224161999508995,
0.104422493053066));
#22818=CARTESIAN_POINT('Ctrl Pts',(-0.971100730005489,-0.203463743702801,
0.139836317888042));
#22819=CARTESIAN_POINT('Ctrl Pts',(-0.968453058988463,-0.190326085855194,
0.15681442133453));
#22820=CARTESIAN_POINT('Ctrl Pts',(-0.963103647174702,-0.15976606450048,
0.1868781821531));
#22821=CARTESIAN_POINT('Ctrl Pts',(-0.960411259488514,-0.142345102874864,
0.199966927975188));
#22822=CARTESIAN_POINT('Ctrl Pts',(-0.955173119738174,-0.099930567888331,
0.223801617934945));
#22823=CARTESIAN_POINT('Ctrl Pts',(-0.952850216871763,-0.0740444353928835,
0.233157223576061));
#22824=CARTESIAN_POINT('Ctrl Pts',(-0.951592097314,-0.04763,0.238183666596899));
#22825=CARTESIAN_POINT('Origin',(0.,-0.04763,0.));
#22826=CARTESIAN_POINT('',(-0.841298510752802,-0.04763,-0.504455939115715));
#22827=CARTESIAN_POINT('Origin',(0.,-0.04763,0.));
#22828=CARTESIAN_POINT('Origin',(-0.707106781186547,-0.04763,-0.707106781186548));
#22829=CARTESIAN_POINT('Origin',(-0.707106781186547,0.,-0.707106781186548));
#22830=CARTESIAN_POINT('',(-0.504455939115715,-0.04763,-0.841298510752802));
#22831=CARTESIAN_POINT('Ctrl Pts',(-0.504455939115715,-0.04763,-0.841298510752802));
#22832=CARTESIAN_POINT('Ctrl Pts',(-0.508899795931835,-0.0740444353928835,
-0.838633903678357));
#22833=CARTESIAN_POINT('Ctrl Pts',(-0.517157748491652,-0.0999305678883309,
-0.833661031856294));
#22834=CARTESIAN_POINT('Ctrl Pts',(-0.537715343527944,-0.142345102874864,
-0.820511285096538));
#22835=CARTESIAN_POINT('Ctrl Pts',(-0.548874290046456,-0.159766064500479,
-0.813159949759));
#22836=CARTESIAN_POINT('Ctrl Pts',(-0.573915184558107,-0.190326085855194,
-0.795684265985089));
#22837=CARTESIAN_POINT('Ctrl Pts',(-0.587792702767295,-0.203463743702801,
-0.78555112003688));
#22838=CARTESIAN_POINT('Ctrl Pts',(-0.615966552324775,-0.224161999508995,
-0.763642258217233));
#22839=CARTESIAN_POINT('Ctrl Pts',(-0.631684198665438,-0.232861760990032,
-0.750785745543687));
#22840=CARTESIAN_POINT('Ctrl Pts',(-0.663382628119203,-0.244251601209411,
-0.722929908501543));
#22841=CARTESIAN_POINT('Ctrl Pts',(-0.679352081686668,-0.246942143572133,
-0.707917883896095));
#22842=CARTESIAN_POINT('Ctrl Pts',(-0.707917883896095,-0.246942143572133,
-0.679352081686668));
#22843=CARTESIAN_POINT('Ctrl Pts',(-0.722929908501543,-0.244251601209411,
-0.663382628119203));
#22844=CARTESIAN_POINT('Ctrl Pts',(-0.750785745543687,-0.232861760990032,
-0.631684198665439));
#22845=CARTESIAN_POINT('Ctrl Pts',(-0.763642258217232,-0.224161999508995,
-0.615966552324775));
#22846=CARTESIAN_POINT('Ctrl Pts',(-0.78555112003688,-0.203463743702801,
-0.587792702767295));
#22847=CARTESIAN_POINT('Ctrl Pts',(-0.795684265985088,-0.190326085855194,
-0.573915184558107));
#22848=CARTESIAN_POINT('Ctrl Pts',(-0.813159949759,-0.15976606450048,-0.548874290046456));
#22849=CARTESIAN_POINT('Ctrl Pts',(-0.820511285096538,-0.142345102874864,
-0.537715343527944));
#22850=CARTESIAN_POINT('Ctrl Pts',(-0.833661031856294,-0.0999305678883311,
-0.517157748491652));
#22851=CARTESIAN_POINT('Ctrl Pts',(-0.838633903678357,-0.0740444353928836,
-0.508899795931835));
#22852=CARTESIAN_POINT('Ctrl Pts',(-0.841298510752801,-0.04763,-0.504455939115715));
#22853=CARTESIAN_POINT('Origin',(-0.707106781186547,-0.04763,-0.707106781186548));
#22854=CARTESIAN_POINT('Origin',(0.,-0.04763,0.));
#22855=CARTESIAN_POINT('',(-0.238183666596899,-0.04763,-0.951592097314));
#22856=CARTESIAN_POINT('Origin',(0.,-0.04763,0.));
#22857=CARTESIAN_POINT('Origin',(5.55111512312578E-17,-0.04763,-1.));
#22858=CARTESIAN_POINT('Origin',(5.55111512312578E-17,0.,-1.));
#22859=CARTESIAN_POINT('',(0.238183666596899,-0.04763,-0.951592097314));
#22860=CARTESIAN_POINT('Ctrl Pts',(0.238183666596899,-0.04763,-0.951592097314));
#22861=CARTESIAN_POINT('Ctrl Pts',(0.233157223576062,-0.0740444353928835,
-0.952850216871763));
#22862=CARTESIAN_POINT('Ctrl Pts',(0.223801617934946,-0.099930567888331,
-0.955173119738174));
#22863=CARTESIAN_POINT('Ctrl Pts',(0.199966927975188,-0.142345102874864,
-0.960411259488514));
#22864=CARTESIAN_POINT('Ctrl Pts',(0.1868781821531,-0.15976606450048,-0.963103647174702));
#22865=CARTESIAN_POINT('Ctrl Pts',(0.15681442133453,-0.190326085855194,
-0.968453058988463));
#22866=CARTESIAN_POINT('Ctrl Pts',(0.139836317888042,-0.203463743702801,
-0.971100730005489));
#22867=CARTESIAN_POINT('Ctrl Pts',(0.104422493053067,-0.224161999508995,
-0.975530745318961));
#22868=CARTESIAN_POINT('Ctrl Pts',(0.0842175114474173,-0.232861760990032,
-0.977553872336861));
#22869=CARTESIAN_POINT('Ctrl Pts',(0.0421062857595698,-0.244251601209411,
-0.980270995488453));
#22870=CARTESIAN_POINT('Ctrl Pts',(0.0201990724523194,-0.246942143572133,
-0.980948));
#22871=CARTESIAN_POINT('Ctrl Pts',(-0.0201990724523193,-0.246942143572133,
-0.980948));
#22872=CARTESIAN_POINT('Ctrl Pts',(-0.0421062857595697,-0.244251601209411,
-0.980270995488453));
#22873=CARTESIAN_POINT('Ctrl Pts',(-0.0842175114474171,-0.232861760990032,
-0.977553872336861));
#22874=CARTESIAN_POINT('Ctrl Pts',(-0.104422493053067,-0.224161999508995,
-0.975530745318961));
#22875=CARTESIAN_POINT('Ctrl Pts',(-0.139836317888042,-0.203463743702801,
-0.971100730005489));
#22876=CARTESIAN_POINT('Ctrl Pts',(-0.15681442133453,-0.190326085855194,
-0.968453058988463));
#22877=CARTESIAN_POINT('Ctrl Pts',(-0.1868781821531,-0.15976606450048,-0.963103647174702));
#22878=CARTESIAN_POINT('Ctrl Pts',(-0.199966927975188,-0.142345102874864,
-0.960411259488514));
#22879=CARTESIAN_POINT('Ctrl Pts',(-0.223801617934945,-0.099930567888331,
-0.955173119738174));
#22880=CARTESIAN_POINT('Ctrl Pts',(-0.233157223576062,-0.0740444353928835,
-0.952850216871763));
#22881=CARTESIAN_POINT('Ctrl Pts',(-0.238183666596899,-0.0476299999999999,
-0.951592097314));
#22882=CARTESIAN_POINT('Origin',(5.55111512312578E-17,-0.04763,-1.));
#22883=CARTESIAN_POINT('Origin',(0.,-0.04763,0.));
#22884=CARTESIAN_POINT('',(0.504455939115715,-0.04763,-0.841298510752802));
#22885=CARTESIAN_POINT('Origin',(0.,-0.04763,0.));
#22886=CARTESIAN_POINT('Origin',(0.707106781186548,-0.04763,-0.707106781186547));
#22887=CARTESIAN_POINT('Origin',(0.707106781186548,0.,-0.707106781186547));
#22888=CARTESIAN_POINT('',(0.841298510752802,-0.04763,-0.504455939115715));
#22889=CARTESIAN_POINT('Ctrl Pts',(0.841298510752802,-0.04763,-0.504455939115715));
#22890=CARTESIAN_POINT('Ctrl Pts',(0.838633903678357,-0.0740444353928835,
-0.508899795931835));
#22891=CARTESIAN_POINT('Ctrl Pts',(0.833661031856294,-0.0999305678883309,
-0.517157748491652));
#22892=CARTESIAN_POINT('Ctrl Pts',(0.820511285096538,-0.142345102874864,
-0.537715343527944));
#22893=CARTESIAN_POINT('Ctrl Pts',(0.813159949759,-0.159766064500479,-0.548874290046456));
#22894=CARTESIAN_POINT('Ctrl Pts',(0.795684265985088,-0.190326085855194,
-0.573915184558107));
#22895=CARTESIAN_POINT('Ctrl Pts',(0.78555112003688,-0.203463743702801,
-0.587792702767295));
#22896=CARTESIAN_POINT('Ctrl Pts',(0.763642258217233,-0.224161999508995,
-0.615966552324775));
#22897=CARTESIAN_POINT('Ctrl Pts',(0.750785745543687,-0.232861760990032,
-0.631684198665438));
#22898=CARTESIAN_POINT('Ctrl Pts',(0.722929908501543,-0.244251601209411,
-0.663382628119203));
#22899=CARTESIAN_POINT('Ctrl Pts',(0.707917883896095,-0.246942143572133,
-0.679352081686668));
#22900=CARTESIAN_POINT('Ctrl Pts',(0.679352081686668,-0.246942143572133,
-0.707917883896095));
#22901=CARTESIAN_POINT('Ctrl Pts',(0.663382628119203,-0.244251601209411,
-0.722929908501543));
#22902=CARTESIAN_POINT('Ctrl Pts',(0.631684198665438,-0.232861760990032,
-0.750785745543687));
#22903=CARTESIAN_POINT('Ctrl Pts',(0.615966552324775,-0.224161999508995,
-0.763642258217232));
#22904=CARTESIAN_POINT('Ctrl Pts',(0.587792702767295,-0.203463743702801,
-0.78555112003688));
#22905=CARTESIAN_POINT('Ctrl Pts',(0.573915184558107,-0.190326085855194,
-0.795684265985088));
#22906=CARTESIAN_POINT('Ctrl Pts',(0.548874290046456,-0.159766064500479,
-0.813159949759));
#22907=CARTESIAN_POINT('Ctrl Pts',(0.537715343527944,-0.142345102874864,
-0.820511285096538));
#22908=CARTESIAN_POINT('Ctrl Pts',(0.517157748491652,-0.099930567888331,
-0.833661031856294));
#22909=CARTESIAN_POINT('Ctrl Pts',(0.508899795931835,-0.0740444353928835,
-0.838633903678357));
#22910=CARTESIAN_POINT('Ctrl Pts',(0.504455939115715,-0.04763,-0.841298510752801));
#22911=CARTESIAN_POINT('Origin',(0.707106781186548,-0.04763,-0.707106781186547));
#22912=CARTESIAN_POINT('Origin',(0.,-0.166705,0.));
#22913=CARTESIAN_POINT('',(-0.980948,-0.28578,1.20131482833E-16));
#22914=CARTESIAN_POINT('Origin',(0.,-0.28578,0.));
#22915=CARTESIAN_POINT('',(-0.980948,-0.166705,1.20131482833E-16));
#22916=CARTESIAN_POINT('',(0.951592097314,-0.04763,0.238183666596899));
#22917=CARTESIAN_POINT('Origin',(0.,-0.04763,0.));
#22918=CARTESIAN_POINT('',(0.951592097314,-0.04763,-0.238183666596899));
#22919=CARTESIAN_POINT('Ctrl Pts',(0.951592097314,-0.04763,0.238183666596899));
#22920=CARTESIAN_POINT('Ctrl Pts',(0.952850216871763,-0.0740444353928835,
0.233157223576062));
#22921=CARTESIAN_POINT('Ctrl Pts',(0.955173119738174,-0.099930567888331,
0.223801617934945));
#22922=CARTESIAN_POINT('Ctrl Pts',(0.960411259488514,-0.142345102874864,
0.199966927975188));
#22923=CARTESIAN_POINT('Ctrl Pts',(0.963103647174702,-0.15976606450048,
0.1868781821531));
#22924=CARTESIAN_POINT('Ctrl Pts',(0.968453058988463,-0.190326085855194,
0.15681442133453));
#22925=CARTESIAN_POINT('Ctrl Pts',(0.971100730005489,-0.203463743702801,
0.139836317888042));
#22926=CARTESIAN_POINT('Ctrl Pts',(0.975530745318961,-0.224161999508995,
0.104422493053067));
#22927=CARTESIAN_POINT('Ctrl Pts',(0.977553872336861,-0.232861760990032,
0.0842175114474172));
#22928=CARTESIAN_POINT('Ctrl Pts',(0.980270995488453,-0.244251601209411,
0.0421062857595697));
#22929=CARTESIAN_POINT('Ctrl Pts',(0.980948,-0.246942143572133,0.0201990724523194));
#22930=CARTESIAN_POINT('Ctrl Pts',(0.980948,-0.246942143572133,-0.0201990724523194));
#22931=CARTESIAN_POINT('Ctrl Pts',(0.980270995488453,-0.244251601209411,
-0.0421062857595697));
#22932=CARTESIAN_POINT('Ctrl Pts',(0.977553872336861,-0.232861760990032,
-0.0842175114474172));
#22933=CARTESIAN_POINT('Ctrl Pts',(0.975530745318961,-0.224161999508995,
-0.104422493053067));
#22934=CARTESIAN_POINT('Ctrl Pts',(0.971100730005489,-0.203463743702801,
-0.139836317888042));
#22935=CARTESIAN_POINT('Ctrl Pts',(0.968453058988463,-0.190326085855194,
-0.15681442133453));
#22936=CARTESIAN_POINT('Ctrl Pts',(0.963103647174702,-0.15976606450048,
-0.1868781821531));
#22937=CARTESIAN_POINT('Ctrl Pts',(0.960411259488514,-0.142345102874864,
-0.199966927975188));
#22938=CARTESIAN_POINT('Ctrl Pts',(0.955173119738174,-0.099930567888331,
-0.223801617934945));
#22939=CARTESIAN_POINT('Ctrl Pts',(0.952850216871763,-0.0740444353928835,
-0.233157223576062));
#22940=CARTESIAN_POINT('Ctrl Pts',(0.951592097314,-0.0476299999999999,-0.238183666596899));
#22941=CARTESIAN_POINT('Origin',(0.,-0.04763,0.));
#22942=CARTESIAN_POINT('Origin',(0.,-0.04763,0.));
#22943=CARTESIAN_POINT('Origin',(1.,-0.04763,0.));
#22944=CARTESIAN_POINT('Origin',(1.,0.,0.));
#22945=CARTESIAN_POINT('Origin',(1.,-0.04763,0.));
#22946=CARTESIAN_POINT('Origin',(0.,-0.28578,0.));
#22947=CARTESIAN_POINT('Origin',(0.,-0.04763,0.));
#26949=UNCERTAINTY_MEASURE_WITH_UNIT(LENGTH_MEASURE(0.001),#27070,
'DISTANCE_ACCURACY_VALUE',
'Maximum model space distance between geometric entities at asserted c
onnectivities');
#26992=UNCERTAINTY_MEASURE_WITH_UNIT(LENGTH_MEASURE(0.001),#27070,
'DISTANCE_ACCURACY_VALUE',
'Maximum model space distance between geometric entities at asserted c
onnectivities');
#27026=(
GEOMETRIC_REPRESENTATION_CONTEXT(3)
GLOBAL_UNCERTAINTY_ASSIGNED_CONTEXT((#26949))
GLOBAL_UNIT_ASSIGNED_CONTEXT((#27070,#27072,#27073))
REPRESENTATION_CONTEXT('','3D')
);
#27069=(
GEOMETRIC_REPRESENTATION_CONTEXT(3)
GLOBAL_UNCERTAINTY_ASSIGNED_CONTEXT((#26992))
GLOBAL_UNIT_ASSIGNED_CONTEXT((#27070,#27072,#27073))
REPRESENTATION_CONTEXT('','3D')
);
#27070=(
LENGTH_UNIT()
NAMED_UNIT(*)
SI_UNIT(.CENTI.,.METRE.)
);
#27072=(
NAMED_UNIT(*)
PLANE_ANGLE_UNIT()
SI_UNIT($,.RADIAN.)
);
#27073=(
NAMED_UNIT(*)
SI_UNIT($,.STERADIAN.)
SOLID_ANGLE_UNIT()
);
#27107=SHAPE_DEFINITION_REPRESENTATION(#27183,#27384);
#27183=PRODUCT_DEFINITION_SHAPE('',$,#27461);
#27384=SHAPE_REPRESENTATION('',(#15247),#27026);
#27427=PRODUCT_DEFINITION_CONTEXT('part definition',#27657,'design');
#27461=PRODUCT_DEFINITION('Cage','Cage',#27537,#27427);
#27537=PRODUCT_DEFINITION_FORMATION('',$,#27692);
#27657=APPLICATION_CONTEXT(
'Core Data for Automotive Mechanical Design Process');
#27658=PRODUCT_CONTEXT('part definition',#27657,'mechanical');
#27692=PRODUCT('Cage','Cage','Cage',(#27658));
#27791=COLOUR_RGB('Grey',0.48,0.52,0.57);
#27792=FILL_AREA_STYLE_COLOUR('',#27791);
#27793=FILL_AREA_STYLE('',(#27792));
#27794=SURFACE_STYLE_FILL_AREA(#27793);
#27795=SURFACE_SIDE_STYLE('',(#27794));
#27796=SURFACE_STYLE_USAGE(.BOTH.,#27795);
#27797=PRESENTATION_STYLE_ASSIGNMENT((#27796));
ENDSEC;
END-ISO-10303-21;
